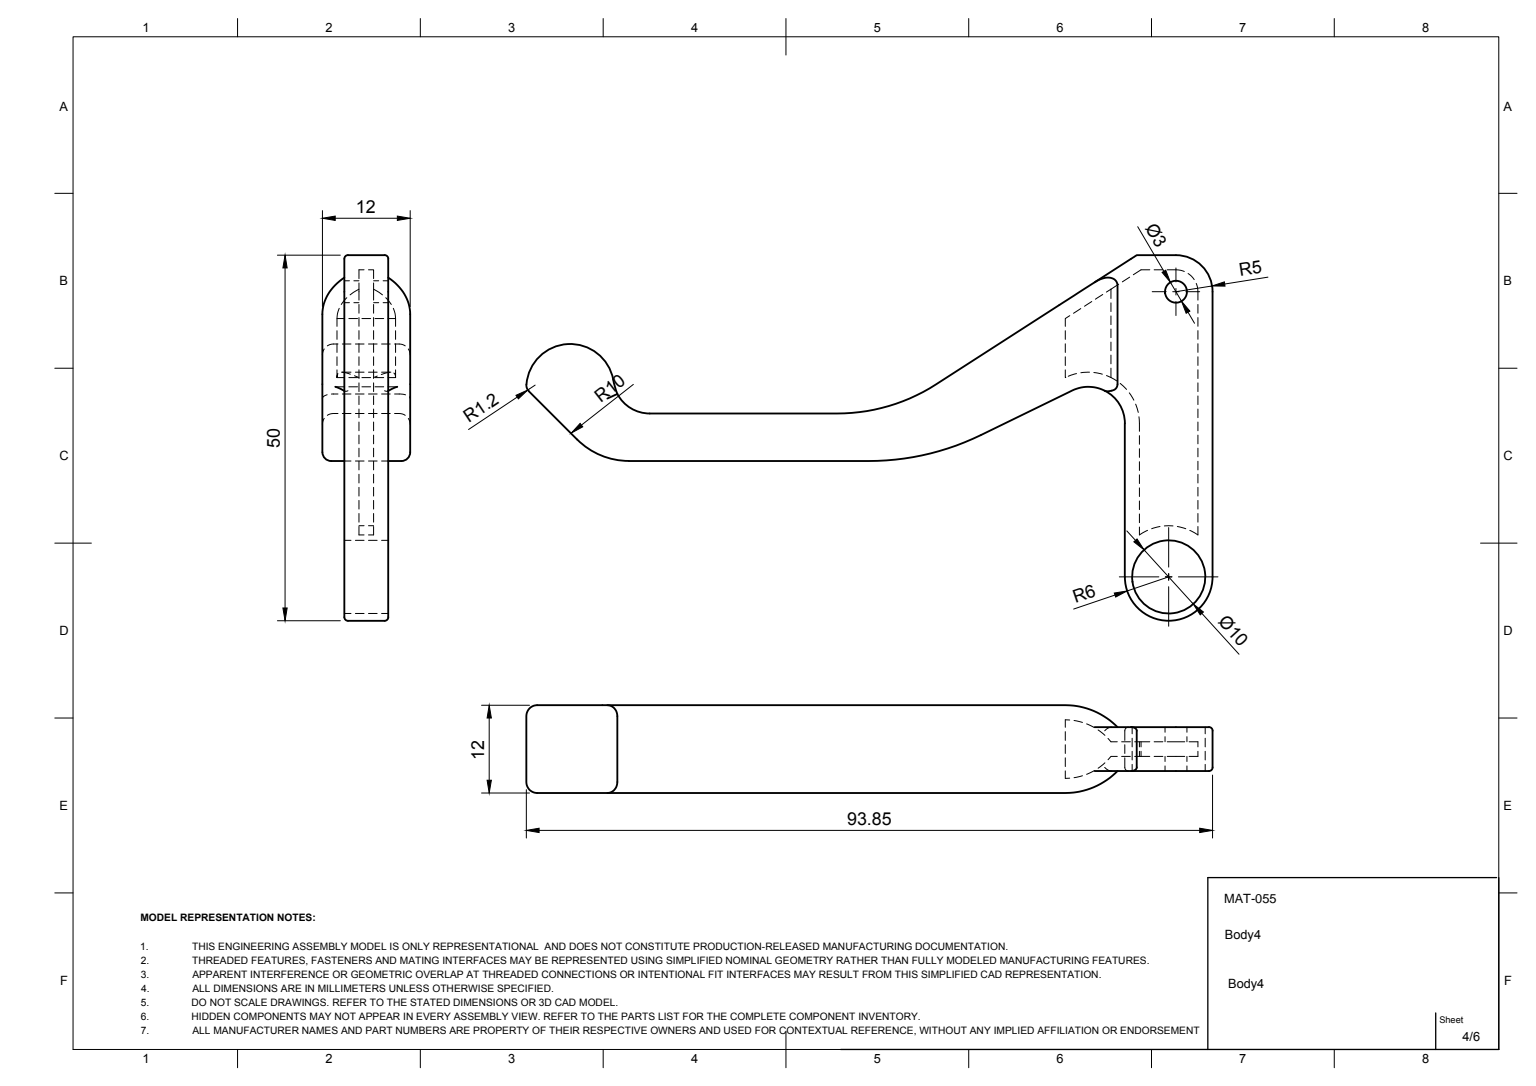
ISO-10303-21;
HEADER;
FILE_DESCRIPTION (('STEP AP214'),
    '1' );
FILE_NAME ('Body4.step',
    '2026-10-30T09:41:00',
    ( '' ),
    ( '' ),
    'SwSTEP 2.0',
    'SolidWorks 2020',
    '' );
FILE_SCHEMA (( 'AUTOMOTIVE_DESIGN' ));
ENDSEC;

DATA;
#3=ORIENTED_EDGE ( 'NONE', *, *, #32082, .F. ) ;
#28=DIRECTION ( 'NONE',  ( 0.000000000000000000, 0.000000000000000000, -1.000000000000000000 ) ) ;
#32=CARTESIAN_POINT ( 'NONE',  ( 74.32979735608419958, -48.45188957854135481, -10.89321520033831447 ) ) ;
#75=ORIENTED_EDGE ( 'NONE', *, *, #33478, .T. ) ;
#76=AXIS2_PLACEMENT_3D ( 'NONE', #7945, #18211, #24609 ) ;
#84=B_SPLINE_CURVE_WITH_KNOTS ( 'NONE', 3,
 ( #40412, #43376, #5506, #23076, #29462, #30146, #44061, #26048, #15786, #12373 ),
 .UNSPECIFIED., .F., .F.,
 ( 4, 2, 2, 2, 4 ),
 ( 0.000000000000000000, 0.0003215953659093761900, 0.0006431907318187523800, 0.0009647860977281285701, 0.001286381463637504760 ),
 .UNSPECIFIED. ) ;
#133=B_SPLINE_CURVE_WITH_KNOTS ( 'NONE', 3,
 ( #26160, #29806, #32757, #36631, #33206, #33421, #5174, #29130, #43042, #26387, #19321, #1981, #18865, #15907, #43720, #40297, #19544, #22961, #9061, #39624, #36853, #40065, #5622, #19092, #8163, #15001, #35960, #8830, #28914, #1530, #42824, #25494, #39398, #32977, #11810 ),
 .UNSPECIFIED., .F., .F.,
 ( 4, 2, 2, 1, 1, 2, 2, 1, 2, 2, 1, 1, 1, 1, 2, 2, 1, 1, 1, 1, 2, 2, 4 ),
 ( 0.000000000000000000, 0.06250000000002535472, 0.1250000000000507094, 0.1875000000000760503, 0.2187500000000859035, 0.2343750000000941469, 0.2500000000001023626, 0.3125000000001353362, 0.3281250000001413869, 0.3437500000001474376, 0.3750000000001494360, 0.4375000000001431633, 0.4687500000001400546, 0.4843750000001384448, 0.4921875000001327272, 0.5000000000001270095, 0.6250000000001643130, 0.6875000000001828537, 0.7187500000001921796, 0.7343750000001968425, 0.7421875000001944001, 0.7500000000001918465, 1.000000000000000000 ),
 .UNSPECIFIED. ) ;
#140=CARTESIAN_POINT ( 'NONE',  ( 63.90572062191856872, -12.84802420451643812, -16.01116961145836370 ) ) ;
#144=DIRECTION ( 'NONE',  ( 0.000000000000000000, 0.000000000000000000, -1.000000000000000000 ) ) ;
#154=CARTESIAN_POINT ( 'NONE',  ( 74.47157298427187300, -3.053873105668316601, -12.39321520033831447 ) ) ;
#166=VERTEX_POINT ( 'NONE', #36740 ) ;
#185=CYLINDRICAL_SURFACE ( 'NONE', #31797, 1.499999999999999556 ) ;
#188=( BOUNDED_CURVE ( )  B_SPLINE_CURVE ( 3, ( #13503, #13725, #28295, #3452 ),
 .UNSPECIFIED., .F., .F. ) 
 B_SPLINE_CURVE_WITH_KNOTS ( ( 4, 4 ),
 ( 4.712388980384689674, 4.721492906269370238 ),
 .UNSPECIFIED. ) 
 CURVE ( )  GEOMETRIC_REPRESENTATION_ITEM ( )  RATIONAL_B_SPLINE_CURVE ( ( 1.000000000000000000, 0.9999930932230500780, 0.9999930932230500780, 1.000000000000000000 ) ) 
 REPRESENTATION_ITEM ( '' )  );
#204=CARTESIAN_POINT ( 'NONE',  ( 70.47992290675011873, 2.032776587329049978, -16.39321520033831447 ) ) ;
#214=CARTESIAN_POINT ( 'NONE',  ( 64.04449450084898388, -15.08552066177155382, -16.37144510805424957 ) ) ;
#215=DIRECTION ( 'NONE',  ( -0.1352586133457950590, -0.9908103287288504424, 0.000000000000000000 ) ) ;
#226=DIRECTION ( 'NONE',  ( 0.000000000000000000, 0.000000000000000000, -1.000000000000000000 ) ) ;
#257=CARTESIAN_POINT ( 'NONE',  ( 64.46696884417693241, -15.35047623415474405, -15.89321305673442986 ) ) ;
#259=VERTEX_POINT ( 'NONE', #5961 ) ;
#276=EDGE_CURVE ( 'NONE', #36610, #20781, #19248, .T. ) ;
#291=CARTESIAN_POINT ( 'NONE',  ( 27.57768543387103222, -14.97172645945875935, -19.39321520033831447 ) ) ;
#293=ORIENTED_EDGE ( 'NONE', *, *, #35379, .F. ) ;
#305=CARTESIAN_POINT ( 'NONE',  ( 74.32979735608419958, -48.45188957854135481, -10.39321520033831625 ) ) ;
#312=ORIENTED_EDGE ( 'NONE', *, *, #19134, .T. ) ;
#326=AXIS2_PLACEMENT_3D ( 'NONE', #2034, #13672, #6599 ) ;
#349=AXIS2_PLACEMENT_3D ( 'NONE', #13047, #20117, #28 ) ;
#362=CARTESIAN_POINT ( 'NONE',  ( 61.78196040322745120, -12.46576002031727448, -17.04883285403948534 ) ) ;
#369=FACE_OUTER_BOUND ( 'NONE', #21979, .T. ) ;
#401=EDGE_CURVE ( 'NONE', #31742, #38280, #42421, .T. ) ;
#430=CIRCLE ( 'NONE', #37583, 1.200000000000000178 ) ;
#432=ORIENTED_EDGE ( 'NONE', *, *, #12226, .F. ) ;
#436=CARTESIAN_POINT ( 'NONE',  ( 62.89921056888596240, -13.37922507188889654, -18.73918694084264303 ) ) ;
#440=AXIS2_PLACEMENT_3D ( 'NONE', #42881, #38535, #14611 ) ;
#469=EDGE_CURVE ( 'NONE', #23752, #259, #6849, .T. ) ;
#472=DIRECTION ( 'NONE',  ( 0.000000000000000000, 0.000000000000000000, -1.000000000000000000 ) ) ;
#478=LINE ( 'NONE', #3232, #42202 ) ;
#490=EDGE_CURVE ( 'NONE', #13961, #15605, #188, .T. ) ;
#497=CARTESIAN_POINT ( 'NONE',  ( 64.24243542014160369, -41.01918285936451269, -16.39321520033831447 ) ) ;
#511=VERTEX_POINT ( 'NONE', #38315 ) ;
#512=AXIS2_PLACEMENT_3D ( 'NONE', #29324, #1497, #9256 ) ;
#522=EDGE_CURVE ( 'NONE', #12356, #39715, #34544, .T. ) ;
#531=DIRECTION ( 'NONE',  ( 0.000000000000000000, 0.000000000000000000, -1.000000000000000000 ) ) ;
#532=ADVANCED_FACE ( 'NONE', ( #3665 ), #7307, .T. ) ;
#553=DIRECTION ( 'NONE',  ( -0.6049664196031393493, 0.7962509850245451659, 0.000000000000000000 ) ) ;
#554=CARTESIAN_POINT ( 'NONE',  ( 62.74499803203641335, -14.59121584191781018, -17.38686684484656908 ) ) ;
#556=EDGE_LOOP ( 'NONE', ( #34925, #21880, #41263, #43526, #26990, #41505, #39389, #13719, #5501, #37121, #24239, #17991 ) ) ;
#560=CARTESIAN_POINT ( 'NONE',  ( 64.90995917204980969, -13.28308322077656278, -11.63059948780157349 ) ) ;
#584=DIRECTION ( 'NONE',  ( 0.000000000000000000, 0.000000000000000000, -1.000000000000000000 ) ) ;
#661=CARTESIAN_POINT ( 'NONE',  ( 64.65529483955577916, -15.48286765530762388, -15.65793769818279735 ) ) ;
#671=CARTESIAN_POINT ( 'NONE',  ( 27.57768543387103222, -14.97172645945875935, -19.39321520033831447 ) ) ;
#677=CARTESIAN_POINT ( 'NONE',  ( 61.14757329627086335, -2.318400467695852285, -17.89321520033712432 ) ) ;
#698=ORIENTED_EDGE ( 'NONE', *, *, #12294, .T. ) ;
#712=CARTESIAN_POINT ( 'NONE',  ( 63.70438564670760684, -13.53232477329181727, -18.38352350030624294 ) ) ;
#716=ORIENTED_EDGE ( 'NONE', *, *, #37812, .T. ) ;
#750=EDGE_LOOP ( 'NONE', ( #41830, #3198, #2175, #16810 ) ) ;
#764=CARTESIAN_POINT ( 'NONE',  ( 35.90261398037149121, 14.17005867477686820, -19.39321520033831447 ) ) ;
#772=CARTESIAN_POINT ( 'NONE',  ( 64.39654352178588681, -13.03842319615433709, -11.15581236813648935 ) ) ;
#788=EDGE_LOOP ( 'NONE', ( #32650, #7157 ) ) ;
#799=CARTESIAN_POINT ( 'NONE',  ( 64.46696884418977902, -15.35047623416358142, -10.89321734395795893 ) ) ;
#809=DIRECTION ( 'NONE',  ( -0.1352586133457901185, -0.9908103287288512195, 0.000000000000000000 ) ) ;
#810=AXIS2_PLACEMENT_3D ( 'NONE', #14418, #28328, #11900 ) ;
#812=CARTESIAN_POINT ( 'NONE',  ( 60.96717296766336602, -14.49347760901631688, -8.701126109306295930 ) ) ;
#854=VERTEX_POINT ( 'NONE', #33717 ) ;
#857=EDGE_CURVE ( 'NONE', #16139, #18111, #18527, .T. ) ;
#873=VERTEX_POINT ( 'NONE', #7043 ) ;
#880=CARTESIAN_POINT ( 'NONE',  ( 59.41476255453773803, -13.68180535374018092, -7.393215200338314474 ) ) ;
#898=DIRECTION ( 'NONE',  ( 0.000000000000000000, 0.000000000000000000, 1.000000000000000000 ) ) ;
#905=CARTESIAN_POINT ( 'NONE',  ( 61.98291279206183191, -3.705398587646214992, -19.39321520033831447 ) ) ;
#915=DIRECTION ( 'NONE',  ( 0.9908103287288504424, -0.1352586133457951423, 0.000000000000000000 ) ) ;
#932=CARTESIAN_POINT ( 'NONE',  ( -1.145390592550938447, -14.88589425535891841, -7.393215200338315363 ) ) ;
#938=EDGE_LOOP ( 'NONE', ( #22426, #35188, #1636, #40965 ) ) ;
#944=CARTESIAN_POINT ( 'NONE',  ( 66.31928500851137187, -14.71576354012722021, -16.39321520033831447 ) ) ;
#1006=CARTESIAN_POINT ( 'NONE',  ( -1.637506834317598026, -6.775152287193681566, -8.893215200338314474 ) ) ;
#1035=EDGE_CURVE ( 'NONE', #40192, #37616, #36694, .T. ) ;
#1037=CARTESIAN_POINT ( 'NONE',  ( 64.06711464991177252, -13.62989902061672431, -8.594543081115894267 ) ) ;
#1043=DIRECTION ( 'NONE',  ( 0.000000000000000000, 0.000000000000000000, -1.000000000000000000 ) ) ;
#1064=ADVANCED_FACE ( 'NONE', ( #14107 ), #43297, .T. ) ;
#1067=CARTESIAN_POINT ( 'NONE',  ( 65.10287265247757205, -0.4742552606671820992, -16.39321520033831447 ) ) ;
#1079=ORIENTED_EDGE ( 'NONE', *, *, #19134, .F. ) ;
#1083=CARTESIAN_POINT ( 'NONE',  ( 80.41643495664496299, -3.865424785743087899, -10.39321520033831625 ) ) ;
#1084=CARTESIAN_POINT ( 'NONE',  ( 64.05455464101120810, -2.913905561056498339, -7.947895114335570277 ) ) ;
#1111=CARTESIAN_POINT ( 'NONE',  ( 63.72671350766138687, -14.88170162854069645, -18.28103043643234571 ) ) ;
#1126=LINE ( 'NONE', #14821, #18340 ) ;
#1143=CARTESIAN_POINT ( 'NONE',  ( 53.69308256885118169, -7.449060273445263114, -7.393215200338315363 ) ) ;
#1144=DIRECTION ( 'NONE',  ( 0.1352586133457901185, 0.9908103287288512195, 0.000000000000000000 ) ) ;
#1145=VECTOR ( 'NONE', #26126, 999.9999999999998863 ) ;
#1153=ORIENTED_EDGE ( 'NONE', *, *, #29788, .T. ) ;
#1169=CIRCLE ( 'NONE', #19398, 10.00000000000000000 ) ;
#1173=ORIENTED_EDGE ( 'NONE', *, *, #20334, .T. ) ;
#1191=CARTESIAN_POINT ( 'NONE',  ( 64.46696884418977902, -15.35047623416358142, -10.89321734395795893 ) ) ;
#1195=ORIENTED_EDGE ( 'NONE', *, *, #29638, .F. ) ;
#1199=DIRECTION ( 'NONE',  ( 0.000000000000000000, 0.000000000000000000, 1.000000000000000000 ) ) ;
#1203=CARTESIAN_POINT ( 'NONE',  ( 0.04488520489200759078, -6.166763362545027327, -18.19321520033831519 ) ) ;
#1211=ORIENTED_EDGE ( 'NONE', *, *, #8860, .T. ) ;
#1213=DIRECTION ( 'NONE',  ( -0.1352586133457950590, -0.9908103287288504424, 0.000000000000000000 ) ) ;
#1228=ORIENTED_EDGE ( 'NONE', *, *, #14201, .T. ) ;
#1261=AXIS2_PLACEMENT_3D ( 'NONE', #32042, #144, #7420 ) ;
#1263=DIRECTION ( 'NONE',  ( 0.000000000000000000, 0.000000000000000000, 1.000000000000000000 ) ) ;
#1265=CARTESIAN_POINT ( 'NONE',  ( 62.93954589823548673, -14.63888995810886051, -9.517290379660753530 ) ) ;
#1283=CIRCLE ( 'NONE', #23133, 1.499999999999998002 ) ;
#1285=CARTESIAN_POINT ( 'NONE',  ( -13.48289411298945595, -4.891473392625994343, -19.20673326947127180 ) ) ;
#1292=ORIENTED_EDGE ( 'NONE', *, *, #34484, .F. ) ;
#1293=CARTESIAN_POINT ( 'NONE',  ( 80.41643495664496299, -3.865424785743087899, -10.89321520033831447 ) ) ;
#1308=CARTESIAN_POINT ( 'NONE',  ( -13.00275943959160685, -4.132914642980755282, -7.537981892864975109 ) ) ;
#1314=EDGE_CURVE ( 'NONE', #7942, #42460, #4050, .T. ) ;
#1317=CARTESIAN_POINT ( 'NONE',  ( 65.55689610126231059, -13.67296395165911704, -12.39321520033831447 ) ) ;
#1330=CARTESIAN_POINT ( 'NONE',  ( 59.24641515291911986, -13.72835195454734425, -7.393215200338315363 ) ) ;
#1343=FILL_AREA_STYLE_COLOUR ( '', #11399 ) ;
#1353=EDGE_LOOP ( 'NONE', ( #6893, #31759, #18475, #18995, #18699 ) ) ;
#1370=CARTESIAN_POINT ( 'NONE',  ( 59.36680634945873436, -12.84644995903807541, -9.393215200338314474 ) ) ;
#1376=ORIENTED_EDGE ( 'NONE', *, *, #23481, .F. ) ;
#1397=CARTESIAN_POINT ( 'NONE',  ( 75.95778847736514194, -3.256761025687008537, -10.39321520033831625 ) ) ;
#1405=ORIENTED_EDGE ( 'NONE', *, *, #32534, .F. ) ;
#1407=CARTESIAN_POINT ( 'NONE',  ( 75.95778847736514194, -3.256761025687008537, -15.89321520033831447 ) ) ;
#1415=DIRECTION ( 'NONE',  ( 0.000000000000000000, 0.000000000000000000, 1.000000000000000000 ) ) ;
#1417=ORIENTED_EDGE ( 'NONE', *, *, #29638, .T. ) ;
#1426=DIRECTION ( 'NONE',  ( 0.000000000000000000, 0.000000000000000000, 1.000000000000000000 ) ) ;
#1427=ORIENTED_EDGE ( 'NONE', *, *, #41467, .F. ) ;
#1446=AXIS2_PLACEMENT_3D ( 'NONE', #14470, #25412, #11053 ) ;
#1469=VECTOR ( 'NONE', #21811, 1000.000000000000114 ) ;
#1483=CARTESIAN_POINT ( 'NONE',  ( 65.55342193993762123, -16.16218099987542800, -9.830679638262655118 ) ) ;
#1488=CARTESIAN_POINT ( 'NONE',  ( 66.31928500851137187, -14.71576354012722021, -10.39321520033831625 ) ) ;
#1497=DIRECTION ( 'NONE',  ( 0.000000000000000000, 0.000000000000000000, -1.000000000000000000 ) ) ;
#1498=VECTOR ( 'NONE', #3951, 1000.000000000000000 ) ;
#1527=CARTESIAN_POINT ( 'NONE',  ( 68.14371629974728251, -1.351251493923715685, -10.39321520033831625 ) ) ;
#1530=CARTESIAN_POINT ( 'NONE',  ( 66.05753635973103144, -0.1399854074271419946, -16.39321520033832158 ) ) ;
#1571=FACE_OUTER_BOUND ( 'NONE', #24276, .T. ) ;
#1591=CARTESIAN_POINT ( 'NONE',  ( 66.31928500851137187, -14.71576354012722021, -16.39321520033831447 ) ) ;
#1611=EDGE_LOOP ( 'NONE', ( #21835, #10008, #36290, #40632 ) ) ;
#1620=ORIENTED_EDGE ( 'NONE', *, *, #9988, .T. ) ;
#1626=VERTEX_POINT ( 'NONE', #1984 ) ;
#1632=CIRCLE ( 'NONE', #25668, 7.000000000000000888 ) ;
#1636=ORIENTED_EDGE ( 'NONE', *, *, #10913, .F. ) ;
#1667=CARTESIAN_POINT ( 'NONE',  ( -2.527712056240301930, -7.043022739214354289, -7.506402576757856160 ) ) ;
#1683=ORIENTED_EDGE ( 'NONE', *, *, #31150, .F. ) ;
#1687=AXIS2_PLACEMENT_3D ( 'NONE', #22360, #36254, #7999 ) ;
#1705=LINE ( 'NONE', #25445, #8559 ) ;
#1706=CARTESIAN_POINT ( 'NONE',  ( 66.18166293637838749, -0.1100759832042771530, -10.39321520033831625 ) ) ;
#1707=CARTESIAN_POINT ( 'NONE',  ( -1.923444331009816155, -6.861511549474196947, -18.79244370401574216 ) ) ;
#1708=CARTESIAN_POINT ( 'NONE',  ( 65.24959551893836363, -14.08404458135745152, -9.384265616240702101 ) ) ;
#1722=DIRECTION ( 'NONE',  ( 0.9498278979187094739, 0.3127730236694427068, -0.000000000000000000 ) ) ;
#1747=CLOSED_SHELL ( 'NONE', ( #4152, #37866, #40832, #17245, #16199, #21143, #36527, #26583, #23655, #20308, #38149, #18533, #35581, #9060, #4115, #13887, #44627, #15699, #28669, #35867, #21510, #34238, #35882, #34304, #5814, #38233, #42050, #33081, #39264, #10525, #29766, #20277, #13735, #40925, #19555, #43598, #6488, #4374, #15680, #7071, #24586, #1064, #38417, #19728, #39940, #41099, #4945, #44561, #38547, #4966, #20625, #26823, #10638, #12784, #14728, #37236, #36466, #14740, #3572, #33654, #43377, #17043, #18627, #23403, #28076, #37922, #4151, #25624, #14144, #30621, #36573, #2068, #37329, #6478, #6539, #28402, #39232, #44240, #532, #16742, #12305, #32549, #31783, #4091, #35680 ) ) ;
#1795=VERTEX_POINT ( 'NONE', #41877 ) ;
#1833=VECTOR ( 'NONE', #22228, 1000.000000000000000 ) ;
#1884=CARTESIAN_POINT ( 'NONE',  ( 62.60955873541980310, -3.465946903308488647, -19.20240821814916288 ) ) ;
#1885=CARTESIAN_POINT ( 'NONE',  ( -6.962123463324031647, -11.49046785505262136, -19.39321520033831447 ) ) ;
#1912=( BOUNDED_CURVE ( )  B_SPLINE_CURVE ( 3, ( #16184, #40122, #36238, #36461 ),
 .UNSPECIFIED., .F., .F. ) 
 B_SPLINE_CURVE_WITH_KNOTS ( ( 4, 4 ),
 ( 4.664242276651448194, 4.712388980384689674 ),
 .UNSPECIFIED. ) 
 CURVE ( )  GEOMETRIC_REPRESENTATION_ITEM ( )  RATIONAL_B_SPLINE_CURVE ( ( 1.000000000000000000, 0.9998068339056410680, 0.9998068339056410680, 1.000000000000000000 ) ) 
 REPRESENTATION_ITEM ( '' )  );
#1950=CARTESIAN_POINT ( 'NONE',  ( -13.78505786413266243, -3.796669003528118758, -18.12937505555870388 ) ) ;
#1964=CYLINDRICAL_SURFACE ( 'NONE', #9953, 4.999999999999997335 ) ;
#1972=VERTEX_POINT ( 'NONE', #3772 ) ;
#1978=CARTESIAN_POINT ( 'NONE',  ( 62.64330450333520162, -3.453051920597017155, -7.590354665846188453 ) ) ;
#1981=CARTESIAN_POINT ( 'NONE',  ( 67.79734085828376067, -0.4026402971269220643, -16.39321520033831447 ) ) ;
#1984=CARTESIAN_POINT ( 'NONE',  ( 76.63408154409412987, 1.697290617957241565, -10.89321520033831447 ) ) ;
#1993=EDGE_CURVE ( 'NONE', #43140, #12130, #45032, .T. ) ;
#2003=CARTESIAN_POINT ( 'NONE',  ( -12.36826994950264336, -4.374949827406453551, -7.393215200338315363 ) ) ;
#2034=CARTESIAN_POINT ( 'NONE',  ( -1.145390592550938447, -14.88589425535891841, -8.593215200338315540 ) ) ;
#2048=ORIENTED_EDGE ( 'NONE', *, *, #29511, .T. ) ;
#2056=VERTEX_POINT ( 'NONE', #24984 ) ;
#2068=ADVANCED_FACE ( 'NONE', ( #28193 ), #12743, .T. ) ;
#2083=ORIENTED_EDGE ( 'NONE', *, *, #25009, .F. ) ;
#2109=CARTESIAN_POINT ( 'NONE',  ( 62.59689981967161998, -3.470785003659166090, -19.20476018416520958 ) ) ;
#2128=VERTEX_POINT ( 'NONE', #24757 ) ;
#2147=EDGE_CURVE ( 'NONE', #24167, #2128, #34986, .T. ) ;
#2148=CARTESIAN_POINT ( 'NONE',  ( 68.16708570727516303, -1.180063502400580999, -10.39321520033831625 ) ) ;
#2153=ORIENTED_EDGE ( 'NONE', *, *, #14241, .F. ) ;
#2156=CARTESIAN_POINT ( 'NONE',  ( 65.41257106814472877, -15.47412461924279725, -10.39321520033831625 ) ) ;
#2165=FACE_OUTER_BOUND ( 'NONE', #28094, .T. ) ;
#2168=CARTESIAN_POINT ( 'NONE',  ( -13.77941350934472808, -4.501197414032524158, -18.63512858394170379 ) ) ;
#2175=ORIENTED_EDGE ( 'NONE', *, *, #19187, .F. ) ;
#2183=ORIENTED_EDGE ( 'NONE', *, *, #32555, .T. ) ;
#2187=EDGE_CURVE ( 'NONE', #4486, #33968, #12023, .T. ) ;
#2200=CARTESIAN_POINT ( 'NONE',  ( -1.932019669644797988, -4.762702382056356321, -17.89321520033831447 ) ) ;
#2232=CARTESIAN_POINT ( 'NONE',  ( -12.36826994950264513, -4.374949827406456215, -19.39321520033831447 ) ) ;
#2239=DIRECTION ( 'NONE',  ( 0.9063289528979890930, 0.4225728684367167087, 0.000000000000000000 ) ) ;
#2263=DIRECTION ( 'NONE',  ( -0.9908103287288503314, 0.1352586133457950868, 0.000000000000000000 ) ) ;
#2271=ORIENTED_EDGE ( 'NONE', *, *, #12226, .T. ) ;
#2343=ORIENTED_EDGE ( 'NONE', *, *, #857, .F. ) ;
#2344=CARTESIAN_POINT ( 'NONE',  ( -2.588851517412736669, -7.061334938601206979, -7.481563165383908753 ) ) ;
#2355=VECTOR ( 'NONE', #41919, 1000.000000000000000 ) ;
#2376=ORIENTED_EDGE ( 'NONE', *, *, #6085, .T. ) ;
#2388=CARTESIAN_POINT ( 'NONE',  ( 74.82520252044861309, -48.51951888521425360, -16.39321520033831447 ) ) ;
#2399=FACE_OUTER_BOUND ( 'NONE', #27872, .T. ) ;
#2440=EDGE_CURVE ( 'NONE', #5770, #22762, #42644, .T. ) ;
#2464=ORIENTED_EDGE ( 'NONE', *, *, #34499, .F. ) ;
#2490=DIRECTION ( 'NONE',  ( 0.9498278979187092519, 0.3127730236694430399, -0.000000000000000000 ) ) ;
#2509=CARTESIAN_POINT ( 'NONE',  ( -3.429934629567074733, -4.841764211284793618, -19.39321520033831447 ) ) ;
#2573=CARTESIAN_POINT ( 'NONE',  ( -2.615402842485104351, -7.069279208319384722, -7.472031487140878170 ) ) ;
#2590=AXIS2_PLACEMENT_3D ( 'NONE', #14721, #584, #27744 ) ;
#2595=AXIS2_PLACEMENT_3D ( 'NONE', #30427, #27464, #13777 ) ;
#2598=CARTESIAN_POINT ( 'NONE',  ( 60.11760374155740294, -14.70486118635416695, -7.429569208445770734 ) ) ;
#2605=DIRECTION ( 'NONE',  ( -0.9063289528979890930, -0.4225728684367167087, 0.000000000000000000 ) ) ;
#2608=DIRECTION ( 'NONE',  ( 0.000000000000000000, 0.000000000000000000, 1.000000000000000000 ) ) ;
#2615=FACE_OUTER_BOUND ( 'NONE', #42287, .T. ) ;
#2622=DIRECTION ( 'NONE',  ( -0.9908103287288504424, 0.1352586133457950313, 0.000000000000000000 ) ) ;
#2631=STYLED_ITEM ( 'NONE', ( #35992 ), #43323 ) ;
#2652=CARTESIAN_POINT ( 'NONE',  ( 71.62928943233082180, 0.3619606153155430217, -12.39321520033831447 ) ) ;
#2665=ORIENTED_EDGE ( 'NONE', *, *, #4911, .T. ) ;
#2707=DIRECTION ( 'NONE',  ( -0.9908103287288504424, 0.1352586133457950313, 0.000000000000000000 ) ) ;
#2714=LINE ( 'NONE', #30534, #38940 ) ;
#2749=VECTOR ( 'NONE', #7883, 1000.000000000000000 ) ;
#2755=ORIENTED_EDGE ( 'NONE', *, *, #6941, .T. ) ;
#2760=EDGE_LOOP ( 'NONE', ( #31215, #432, #27283, #35161 ) ) ;
#2773=DIRECTION ( 'NONE',  ( 0.000000000000000000, 0.000000000000000000, 1.000000000000000000 ) ) ;
#2786=CARTESIAN_POINT ( 'NONE',  ( 46.47434218039879283, -17.93412427487546523, -8.593215200338315540 ) ) ;
#2787=FACE_OUTER_BOUND ( 'NONE', #19625, .T. ) ;
#2803=ORIENTED_EDGE ( 'NONE', *, *, #25009, .T. ) ;
#2818=VERTEX_POINT ( 'NONE', #291 ) ;
#2850=DIRECTION ( 'NONE',  ( 0.3127730236694482580, -0.9498278979187074755, 0.000000000000000000 ) ) ;
#2852=DIRECTION ( 'NONE',  ( -0.000000000000000000, -0.000000000000000000, 1.000000000000000000 ) ) ;
#2856=CARTESIAN_POINT ( 'NONE',  ( 31.16203868753470019, 11.28474725185576055, -17.89321520033831447 ) ) ;
#2883=CARTESIAN_POINT ( 'NONE',  ( 66.07656475110815109, -2.141145020708993929, -8.744744089885024607 ) ) ;
#2925=AXIS2_PLACEMENT_3D ( 'NONE', #18987, #8724, #11703 ) ;
#2926=CARTESIAN_POINT ( 'NONE',  ( 61.63318325272354770, -19.46990085680238636, -15.89321520033831447 ) ) ;
#2979=DIRECTION ( 'NONE',  ( 0.000000000000000000, 0.000000000000000000, 1.000000000000000000 ) ) ;
#2987=VERTEX_POINT ( 'NONE', #17847 ) ;
#2990=CARTESIAN_POINT ( 'NONE',  ( 61.36049780884140148, -12.47513267055688502, -9.628222199120516578 ) ) ;
#2994=EDGE_CURVE ( 'NONE', #9021, #11150, #41201, .T. ) ;
#2996=EDGE_LOOP ( 'NONE', ( #25071, #25421, #35320, #36704, #2153 ) ) ;
#3010=DIRECTION ( 'NONE',  ( -0.9908103287288505534, 0.1352586133457950035, 0.000000000000000000 ) ) ;
#3046=CIRCLE ( 'NONE', #31438, 26.50000000000000000 ) ;
#3110=CARTESIAN_POINT ( 'NONE',  ( 67.28387040543748299, -1.679813135375296529, -9.537078095872010053 ) ) ;
#3183=VERTEX_POINT ( 'NONE', #42918 ) ;
#3198=ORIENTED_EDGE ( 'NONE', *, *, #522, .F. ) ;
#3222=DIRECTION ( 'NONE',  ( 0.000000000000000000, 0.000000000000000000, 1.000000000000000000 ) ) ;
#3232=CARTESIAN_POINT ( 'NONE',  ( 66.58723489636778936, -20.14619392353143112, -19.39321520033831447 ) ) ;
#3242=ORIENTED_EDGE ( 'NONE', *, *, #6941, .F. ) ;
#3254=CARTESIAN_POINT ( 'NONE',  ( 77.44400397045842510, -3.459648945705700473, -14.39321520033831625 ) ) ;
#3269=ORIENTED_EDGE ( 'NONE', *, *, #25124, .T. ) ;
#3279=CARTESIAN_POINT ( 'NONE',  ( 63.09505974864278244, -3.280483143683338820, -7.685112946281191348 ) ) ;
#3291=CARTESIAN_POINT ( 'NONE',  ( -3.049772195457630897, -7.199189612102626867, -19.39321520033830737 ) ) ;
#3340=CARTESIAN_POINT ( 'NONE',  ( 70.47992290675011873, 2.032776587329049978, -10.39321520033831625 ) ) ;
#3342=CARTESIAN_POINT ( 'NONE',  ( 61.06105367438289733, -12.49321934622164321, -17.22529996229299343 ) ) ;
#3348=DIRECTION ( 'NONE',  ( 0.000000000000000000, 0.000000000000000000, 1.000000000000000000 ) ) ;
#3370=DIRECTION ( 'NONE',  ( -0.000000000000000000, -0.000000000000000000, 1.000000000000000000 ) ) ;
#3373=ORIENTED_EDGE ( 'NONE', *, *, #39824, .F. ) ;
#3386=VERTEX_POINT ( 'NONE', #34336 ) ;
#3388=AXIS2_PLACEMENT_3D ( 'NONE', #28349, #7591, #31979 ) ;
#3389=DIRECTION ( 'NONE',  ( 0.000000000000000000, 0.000000000000000000, 1.000000000000000000 ) ) ;
#3393=CARTESIAN_POINT ( 'NONE',  ( -13.78505786849335379, -3.796669023459796843, -8.893215200338350002 ) ) ;
#3435=AXIS2_PLACEMENT_3D ( 'NONE', #1407, #18297, #4828 ) ;
#3452=CARTESIAN_POINT ( 'NONE',  ( 59.44377208703740223, -12.82110557137145967, -17.39288367676203606 ) ) ;
#3455=DIRECTION ( 'NONE',  ( 0.000000000000000000, 0.000000000000000000, -1.000000000000000000 ) ) ;
#3501=FACE_OUTER_BOUND ( 'NONE', #32187, .T. ) ;
#3548=CARTESIAN_POINT ( 'NONE',  ( 65.70869026611384811, -0.1917948075113792838, -10.71553487254586656 ) ) ;
#3554=CYLINDRICAL_SURFACE ( 'NONE', #2590, 1.499999999999998002 ) ;
#3557=CARTESIAN_POINT ( 'NONE',  ( 63.16361418624702395, -12.63457483197140085, -16.47427386053546527 ) ) ;
#3562=CYLINDRICAL_SURFACE ( 'NONE', #26727, 1.199999999999996625 ) ;
#3568=DIRECTION ( 'NONE',  ( 0.000000000000000000, 0.000000000000000000, -1.000000000000000000 ) ) ;
#3572=ADVANCED_FACE ( 'NONE', ( #11749 ), #21101, .F. ) ;
#3632=CARTESIAN_POINT ( 'NONE',  ( 63.78480611294602909, -13.55202615601718463, -18.34317296867338598 ) ) ;
#3645=FACE_OUTER_BOUND ( 'NONE', #37899, .T. ) ;
#3663=VECTOR ( 'NONE', #42879, 1000.000000000000000 ) ;
#3665=FACE_OUTER_BOUND ( 'NONE', #19411, .T. ) ;
#3668=CARTESIAN_POINT ( 'NONE',  ( 76.56645223742121686, 1.201885453592819397, -10.89321520033831447 ) ) ;
#3676=EDGE_CURVE ( 'NONE', #43140, #23633, #26628, .T. ) ;
#3718=DIRECTION ( 'NONE',  ( -0.9908103287288504424, 0.1352586133457951423, 0.000000000000000000 ) ) ;
#3739=CARTESIAN_POINT ( 'NONE',  ( 63.28220228970403127, -14.74607418324612418, -17.03279905538827066 ) ) ;
#3756=VECTOR ( 'NONE', #13524, 1000.000000000000000 ) ;
#3760=ORIENTED_EDGE ( 'NONE', *, *, #13500, .T. ) ;
#3772=CARTESIAN_POINT ( 'NONE',  ( 76.56645223742121686, 1.201885453592819397, -16.39321520033831447 ) ) ;
#3812=VECTOR ( 'NONE', #10685, 1000.000000000000000 ) ;
#3828=B_SPLINE_CURVE_WITH_KNOTS ( 'NONE', 3,
 ( #11759, #25669, #39574, #18818, #22237, #36357, #1707, #26112, #11988, #25889, #32709, #39794, #5128, #19045, #15630, #29534, #43450, #40018, #22688, #36586, #5361, #27477, #33841, #41396, #30213, #43901, #9694, #3291, #37032 ),
 .UNSPECIFIED., .F., .F.,
 ( 4, 2, 2, 2, 1, 1, 2, 2, 2, 2, 1, 1, 1, 2, 2, 2, 4 ),
 ( 0.000000000000000000, 0.2500000000000469624, 0.3750000000000684452, 0.4375000000000791589, 0.4687500000000845435, 0.4843750000000872080, 0.4921875000000887623, 0.5000000000000902611, 0.6250000000000713873, 0.6875000000000619504, 0.7187500000000581757, 0.7343750000000563993, 0.7421875000000554001, 0.7460937500000548450, 0.7500000000000544009, 0.8750000000000272005, 1.000000000000000000 ),
 .UNSPECIFIED. ) ;
#3830=CARTESIAN_POINT ( 'NONE',  ( 75.95778847736514194, -3.256761025687008537, -10.89321520033831447 ) ) ;
#3854=PLANE ( 'NONE',  #8272 ) ;
#3868=AXIS2_PLACEMENT_3D ( 'NONE', #37031, #2608, #12668 ) ;
#3869=EDGE_CURVE ( 'NONE', #12923, #2818, #28104, .T. ) ;
#3886=DIRECTION ( 'NONE',  ( -0.6049664196031392382, 0.7962509850245451659, 0.000000000000000000 ) ) ;
#3897=MECHANICAL_DESIGN_GEOMETRIC_PRESENTATION_REPRESENTATION('',(#25756),#36635);
#3898=DIRECTION ( 'NONE',  ( -0.9908103287288504424, 0.1352586133457950590, 0.000000000000000000 ) ) ;
#3900=AXIS2_PLACEMENT_3D ( 'NONE', #13422, #23911, #30507 ) ;
#3939=ORIENTED_EDGE ( 'NONE', *, *, #36160, .T. ) ;
#3951=DIRECTION ( 'NONE',  ( -0.9908103287288505534, 0.1352586133457944206, 0.000000000000000000 ) ) ;
#3969=CARTESIAN_POINT ( 'NONE',  ( 65.03532339491583514, -13.35226529162342501, -11.76448087493823280 ) ) ;
#3979=CARTESIAN_POINT ( 'NONE',  ( 54.86886719809545809, -45.79521720516596872, -9.393215200338314474 ) ) ;
#3982=VERTEX_POINT ( 'NONE', #6256 ) ;
#3989=CARTESIAN_POINT ( 'NONE',  ( 60.45894907855897316, -4.846173528048923096, -17.39321520033831447 ) ) ;
#3996=CARTESIAN_POINT ( 'NONE',  ( 62.56397285973651634, -12.53174821361586488, -16.75792485075395533 ) ) ;
#4050=LINE ( 'NONE', #14552, #35258 ) ;
#4091=ADVANCED_FACE ( 'NONE', ( #17201 ), #10993, .T. ) ;
#4092=DIRECTION ( 'NONE',  ( -0.9908103287288503314, 0.1352586133457958362, 0.000000000000000000 ) ) ;
#4107=CARTESIAN_POINT ( 'NONE',  ( 69.69189222815028018, -41.76310523276638520, -10.39321520033831625 ) ) ;
#4115=ADVANCED_FACE ( 'NONE', ( #3501 ), #13551, .T. ) ;
#4151=ADVANCED_FACE ( 'NONE', ( #40928 ), #23597, .F. ) ;
#4152=ADVANCED_FACE ( 'NONE', ( #31760 ), #17638, .F. ) ;
#4153=CARTESIAN_POINT ( 'NONE',  ( 31.16203868753470019, 11.28474725185576055, -7.393215200338315363 ) ) ;
#4167=ORIENTED_EDGE ( 'NONE', *, *, #42868, .F. ) ;
#4189=CARTESIAN_POINT ( 'NONE',  ( 61.41189896420279837, -3.923951091603942398, -19.36498282264282977 ) ) ;
#4210=CIRCLE ( 'NONE', #13702, 0.5000000000000004441 ) ;
#4228=FACE_OUTER_BOUND ( 'NONE', #43371, .T. ) ;
#4230=CARTESIAN_POINT ( 'NONE',  ( 62.22094884293999684, -14.48605613577975681, -7.865232863873874436 ) ) ;
#4236=CYLINDRICAL_SURFACE ( 'NONE', #29693, 8.000000000000000000 ) ;
#4240=EDGE_CURVE ( 'NONE', #17567, #15954, #18311, .T. ) ;
#4258=EDGE_CURVE ( 'NONE', #31347, #23752, #21505, .T. ) ;
#4273=CARTESIAN_POINT ( 'NONE',  ( -13.35201667389344315, -5.063733019641336597, -8.593215170849799023 ) ) ;
#4297=CARTESIAN_POINT ( 'NONE',  ( 75.95778847736514194, -3.256761025687008537, -15.89321520033831447 ) ) ;
#4301=CARTESIAN_POINT ( 'NONE',  ( 62.73786426684350204, -14.56780133514543607, -18.73718775869126318 ) ) ;
#4315=DIRECTION ( 'NONE',  ( -0.9908103287288504424, 0.1352586133457950590, 0.000000000000000000 ) ) ;
#4329=AXIS2_PLACEMENT_3D ( 'NONE', #27418, #40644, #20352 ) ;
#4343=CARTESIAN_POINT ( 'NONE',  ( 65.22669769703878728, -15.48412439713661648, -16.39321520033832513 ) ) ;
#4348=DIRECTION ( 'NONE',  ( -0.9908103287288503314, 0.1352586133457956419, 0.000000000000000000 ) ) ;
#4374=ADVANCED_FACE ( 'NONE', ( #18086 ), #31048, .T. ) ;
#4426=CARTESIAN_POINT ( 'NONE',  ( 63.41431291788855873, -12.69930909095325511, -10.45796961699282690 ) ) ;
#4434=ORIENTED_EDGE ( 'NONE', *, *, #42420, .T. ) ;
#4447=CARTESIAN_POINT ( 'NONE',  ( 60.45894907855897316, -4.846173528048923096, -9.393215200338314474 ) ) ;
#4454=EDGE_CURVE ( 'NONE', #16401, #39949, #1169, .T. ) ;
#4461=CARTESIAN_POINT ( 'NONE',  ( 63.72678816918493538, -14.88173340316315674, -8.505439947836993753 ) ) ;
#4486=VERTEX_POINT ( 'NONE', #20062 ) ;
#4490=SHAPE_DEFINITION_REPRESENTATION ( #14670, #30918 ) ;
#4505=CARTESIAN_POINT ( 'NONE',  ( 66.00964506737828685, -2.167441154595251440, -8.806695022995075561 ) ) ;
#4525=DIRECTION ( 'NONE',  ( 0.000000000000000000, 0.000000000000000000, -1.000000000000000000 ) ) ;
#4532=CARTESIAN_POINT ( 'NONE',  ( 60.62025573688512736, -14.54431086544325247, -19.30358038137204701 ) ) ;
#4542=PLANE ( 'NONE',  #35390 ) ;
#4547=CARTESIAN_POINT ( 'NONE',  ( 67.28358753636723577, -1.679921224420888981, -17.24955508517946967 ) ) ;
#4548=ORIENTED_EDGE ( 'NONE', *, *, #18053, .T. ) ;
#4584=CARTESIAN_POINT ( 'NONE',  ( 65.24959551893836363, -14.08404458135744797, -17.40216478443592507 ) ) ;
#4592=CIRCLE ( 'NONE', #1687, 4.999999999999997335 ) ;
#4613=CARTESIAN_POINT ( 'NONE',  ( 3.060777270043529619, -5.064559853354640317, -8.893215200338314474 ) ) ;
#4623=DIRECTION ( 'NONE',  ( 0.000000000000000000, 0.000000000000000000, -1.000000000000000000 ) ) ;
#4638=DIRECTION ( 'NONE',  ( 0.000000000000000000, 0.000000000000000000, 1.000000000000000000 ) ) ;
#4664=CARTESIAN_POINT ( 'NONE',  ( 60.06931813437629586, -14.72076136720887085, -8.603412892520118760 ) ) ;
#4665=DIRECTION ( 'NONE',  ( 0.9908103287288504424, -0.1352586133457949757, 0.000000000000000000 ) ) ;
#4672=CARTESIAN_POINT ( 'NONE',  ( -13.74784922440762713, -3.813634959067930819, -8.495864720811209025 ) ) ;
#4678=CARTESIAN_POINT ( 'NONE',  ( 66.01387875770896585, -14.50705293059987788, -10.06447537375617252 ) ) ;
#4707=EDGE_LOOP ( 'NONE', ( #16154, #4167, #4930, #15408 ) ) ;
#4744=VERTEX_POINT ( 'NONE', #15891 ) ;
#4755=EDGE_CURVE ( 'NONE', #31560, #2818, #7969, .T. ) ;
#4756=CARTESIAN_POINT ( 'NONE',  ( 55.68041887817022939, -39.85035523279287162, -17.39321520033831447 ) ) ;
#4763=SHAPE_REPRESENTATION_RELATIONSHIP ( 'NONE' , 'NONE' ,  #30918, #43323 ) ;
#4773=EDGE_LOOP ( 'NONE', ( #8065, #43824, #9275, #22865, #23073, #33451 ) ) ;
#4787=DIRECTION ( 'NONE',  ( 1.000000000000000000, 0.000000000000000000, 0.000000000000000000 ) ) ;
#4788=DIRECTION ( 'NONE',  ( -0.9908103287288504424, 0.1352586133457950590, 0.000000000000000000 ) ) ;
#4795=ORIENTED_EDGE ( 'NONE', *, *, #23426, .F. ) ;
#4828=DIRECTION ( 'NONE',  ( 0.9908103287288504424, -0.1352586133457951423, 0.000000000000000000 ) ) ;
#4832=AXIS2_PLACEMENT_3D ( 'NONE', #37080, #13836, #6777 ) ;
#4834=ORIENTED_EDGE ( 'NONE', *, *, #2994, .T. ) ;
#4845=EDGE_CURVE ( 'NONE', #35887, #24167, #34676, .T. ) ;
#4851=DIRECTION ( 'NONE',  ( 0.9908103287288504424, -0.1352586133457952533, 0.000000000000000000 ) ) ;
#4855=CARTESIAN_POINT ( 'NONE',  ( 27.78057335388972504, -13.48551096636548330, -19.39321520033831447 ) ) ;
#4885=ORIENTED_EDGE ( 'NONE', *, *, #33887, .T. ) ;
#4892=LINE ( 'NONE', #43891, #29240 ) ;
#4903=CARTESIAN_POINT ( 'NONE',  ( 59.75121349346655109, -13.58877957849837692, -7.404803486908546617 ) ) ;
#4911=EDGE_CURVE ( 'NONE', #11410, #23361, #23047, .T. ) ;
#4930=ORIENTED_EDGE ( 'NONE', *, *, #14554, .F. ) ;
#4943=EDGE_CURVE ( 'NONE', #2128, #10182, #40530, .T. ) ;
#4945=ADVANCED_FACE ( 'NONE', ( #28730 ), #4542, .F. ) ;
#4949=CARTESIAN_POINT ( 'NONE',  ( -13.43092278348643376, -3.953837739881414848, -7.878202387284918728 ) ) ;
#4966=ADVANCED_FACE ( 'NONE', ( #21878 ), #1964, .T. ) ;
#4977=EDGE_LOOP ( 'NONE', ( #14039, #7606, #8265, #14143 ) ) ;
#5061=EDGE_CURVE ( 'NONE', #32385, #9071, #1912, .T. ) ;
#5070=CYLINDRICAL_SURFACE ( 'NONE', #2925, 35.00000000000000711 ) ;
#5071=EDGE_LOOP ( 'NONE', ( #42487, #7890, #19368, #16058 ) ) ;
#5086=CARTESIAN_POINT ( 'NONE',  ( 67.69800074041313565, -1.521566938544754999, -16.82025522485820446 ) ) ;
#5113=DIRECTION ( 'NONE',  ( 1.000000000000000000, 0.000000000000000000, 0.000000000000000000 ) ) ;
#5116=CARTESIAN_POINT ( 'NONE',  ( 65.52504830115719869, -2.484121567297625788, -16.32284768336232261 ) ) ;
#5128=CARTESIAN_POINT ( 'NONE',  ( -2.055500662264778011, -6.901212958611610659, -18.95048905933739292 ) ) ;
#5129=CARTESIAN_POINT ( 'NONE',  ( 63.13224612813447578, -13.41522658373937915, -8.141029825667127184 ) ) ;
#5133=EDGE_LOOP ( 'NONE', ( #40422, #35648, #18943, #41192 ) ) ;
#5147=CARTESIAN_POINT ( 'NONE',  ( -13.83992782281680078, -4.421549056456191451, -18.43133312422856562 ) ) ;
#5154=ORIENTED_EDGE ( 'NONE', *, *, #41746, .F. ) ;
#5155=DIRECTION ( 'NONE',  ( -0.1352586133458019424, -0.9908103287288495542, 0.000000000000000000 ) ) ;
#5174=CARTESIAN_POINT ( 'NONE',  ( 68.03116533996660564, -0.6815855639037916580, -16.39321520033830737 ) ) ;
#5184=ORIENTED_EDGE ( 'NONE', *, *, #36160, .F. ) ;
#5197=CARTESIAN_POINT ( 'NONE',  ( 74.47157298427187300, -3.053873105668316601, -14.39321520033831625 ) ) ;
#5227=CARTESIAN_POINT ( 'NONE',  ( -3.429934629567074733, -4.841764211284793618, -8.893215200338314474 ) ) ;
#5288=CIRCLE ( 'NONE', #30780, 1.499999999999998002 ) ;
#5301=CARTESIAN_POINT ( 'NONE',  ( 35.90261398037149121, 14.17005867477686820, -8.593215200338315540 ) ) ;
#5307=VECTOR ( 'NONE', #35865, 1000.000000000000000 ) ;
#5311=ORIENTED_EDGE ( 'NONE', *, *, #18143, .T. ) ;
#5318=CARTESIAN_POINT ( 'NONE',  ( 54.86886719809545809, -45.79521720516596872, -17.39321520033831447 ) ) ;
#5319=ORIENTED_EDGE ( 'NONE', *, *, #18365, .F. ) ;
#5320=CARTESIAN_POINT ( 'NONE',  ( -2.326236797655081290, -6.982629615722759198, -7.609261158995283658 ) ) ;
#5337=EDGE_LOOP ( 'NONE', ( #2376, #16218, #13316, #13104 ) ) ;
#5339=CIRCLE ( 'NONE', #43231, 1.200000000000000178 ) ;
#5340=AXIS2_PLACEMENT_3D ( 'NONE', #17069, #38457, #38237 ) ;
#5354=CARTESIAN_POINT ( 'NONE',  ( 64.92272412734682518, -13.29087679925527254, -15.14070786268923285 ) ) ;
#5360=CARTESIAN_POINT ( 'NONE',  ( 67.43171844381110702, -0.1877862098377165168, -10.39321520033831625 ) ) ;
#5361=CARTESIAN_POINT ( 'NONE',  ( -2.501350073892645298, -7.035121566246528069, -19.26840662495741796 ) ) ;
#5375=DIRECTION ( 'NONE',  ( 0.000000000000000000, 0.000000000000000000, -1.000000000000000000 ) ) ;
#5378=CARTESIAN_POINT ( 'NONE',  ( -13.54490672864917045, -3.903797476764282681, -18.73945354926143736 ) ) ;
#5402=CARTESIAN_POINT ( 'NONE',  ( 62.10612082415807578, -3.658631476800715099, -7.496619392082022770 ) ) ;
#5474=CARTESIAN_POINT ( 'NONE',  ( 2.384484203314607420, -10.01861149699890063, -17.89321520033831447 ) ) ;
#5481=AXIS2_PLACEMENT_3D ( 'NONE', #3668, #41768, #27637 ) ;
#5501=ORIENTED_EDGE ( 'NONE', *, *, #32837, .T. ) ;
#5506=CARTESIAN_POINT ( 'NONE',  ( 65.62646388487864613, -15.45076938567549263, -16.39321520033831447 ) ) ;
#5527=EDGE_CURVE ( 'NONE', #11850, #27501, #44454, .T. ) ;
#5535=CARTESIAN_POINT ( 'NONE',  ( 64.28574602589941378, -2.825497480247340043, -18.75418257877172934 ) ) ;
#5538=CARTESIAN_POINT ( 'NONE',  ( -2.556913038227175416, -7.051771562855549291, -7.494178442794038553 ) ) ;
#5574=CIRCLE ( 'NONE', #38355, 1.199999999999999512 ) ;
#5575=CARTESIAN_POINT ( 'NONE',  ( 67.52182966331936598, -0.2245269270738840806, -10.39321520033831980 ) ) ;
#5593=CARTESIAN_POINT ( 'NONE',  ( -13.53629081928688649, -4.821193161180528541, -18.04471655251912665 ) ) ;
#5622=CARTESIAN_POINT ( 'NONE',  ( 66.99801899372408798, -0.07922336130813037447, -16.39321520033831447 ) ) ;
#5695=EDGE_CURVE ( 'NONE', #12923, #25838, #41270, .T. ) ;
#5699=ORIENTED_EDGE ( 'NONE', *, *, #41219, .F. ) ;
#5701=PLANE ( 'NONE',  #40124 ) ;
#5717=ORIENTED_EDGE ( 'NONE', *, *, #23481, .T. ) ;
#5742=DIRECTION ( 'NONE',  ( 0.000000000000000000, 0.000000000000000000, 1.000000000000000000 ) ) ;
#5754=CARTESIAN_POINT ( 'NONE',  ( 62.61854009670715726, -3.462514682154532952, -19.20073182371810461 ) ) ;
#5770=VERTEX_POINT ( 'NONE', #42150 ) ;
#5786=CARTESIAN_POINT ( 'NONE',  ( 66.58723489636778936, -20.14619392353143112, -19.39321520033831447 ) ) ;
#5790=AXIS2_PLACEMENT_3D ( 'NONE', #42439, #10315, #38108 ) ;
#5800=CARTESIAN_POINT ( 'NONE',  ( 67.42381492657879960, -0.1846631707194854588, -10.39321520033831625 ) ) ;
#5814=ADVANCED_FACE ( 'NONE', ( #38929 ), #185, .T. ) ;
#5819=CARTESIAN_POINT ( 'NONE',  ( -13.88591660730176436, -4.361019060476756692, -18.21192235134802928 ) ) ;
#5874=VERTEX_POINT ( 'NONE', #17969 ) ;
#5880=ORIENTED_EDGE ( 'NONE', *, *, #4755, .T. ) ;
#5906=CIRCLE ( 'NONE', #13116, 6.000000000000000888 ) ;
#5925=TOROIDAL_SURFACE ( 'NONE', #24873, 12.50000000000000000, 1.500000000000000000 ) ;
#5946=ORIENTED_EDGE ( 'NONE', *, *, #24219, .T. ) ;
#5961=CARTESIAN_POINT ( 'NONE',  ( 76.56645223742121686, 1.201885453592819397, -10.39321520033831625 ) ) ;
#5964=CIRCLE ( 'NONE', #30751, 4.999999999999997335 ) ;
#5970=VERTEX_POINT ( 'NONE', #32975 ) ;
#5973=CARTESIAN_POINT ( 'NONE',  ( 67.08264006073221708, -20.21382323020432992, -10.89321520033831447 ) ) ;
#5988=CIRCLE ( 'NONE', #27124, 1.200000000000000844 ) ;
#6004=CIRCLE ( 'NONE', #9666, 4.500000000000000888 ) ;
#6025=CARTESIAN_POINT ( 'NONE',  ( 60.53937939559665438, -4.256997083809236138, -8.893215200338314474 ) ) ;
#6029=CARTESIAN_POINT ( 'NONE',  ( 66.93334766501303079, -0.07218023934172421163, -10.39321520033831803 ) ) ;
#6035=FACE_BOUND ( 'NONE', #28332, .T. ) ;
#6043=CARTESIAN_POINT ( 'NONE',  ( 64.73784058450603140, -41.08681216603740438, -7.393215200338315363 ) ) ;
#6083=AXIS2_PLACEMENT_3D ( 'NONE', #32583, #39442, #4092 ) ;
#6085=EDGE_CURVE ( 'NONE', #25838, #873, #43269, .T. ) ;
#6114=EDGE_CURVE ( 'NONE', #41341, #2056, #43717, .T. ) ;
#6119=VERTEX_POINT ( 'NONE', #39396 ) ;
#6123=DIRECTION ( 'NONE',  ( -0.1352586133457944206, -0.9908103287288505534, 0.000000000000000000 ) ) ;
#6134=DIRECTION ( 'NONE',  ( 0.000000000000000000, 0.000000000000000000, -1.000000000000000000 ) ) ;
#6153=AXIS2_PLACEMENT_3D ( 'NONE', #35103, #3886, #24209 ) ;
#6197=FACE_BOUND ( 'NONE', #15997, .T. ) ;
#6224=AXIS2_PLACEMENT_3D ( 'NONE', #6025, #2605, #24055 ) ;
#6227=CARTESIAN_POINT ( 'NONE',  ( 59.62174278132244609, -14.86814543204979344, -18.19321520033831519 ) ) ;
#6256=CARTESIAN_POINT ( 'NONE',  ( 78.93021946355167984, -3.662536865724447921, -12.39321520033831447 ) ) ;
#6268=FACE_OUTER_BOUND ( 'NONE', #37286, .T. ) ;
#6269=CARTESIAN_POINT ( 'NONE',  ( -7.923679509334008664, -5.078949698970065540, -8.893215200338314474 ) ) ;
#6279=CARTESIAN_POINT ( 'NONE',  ( 0.04488520489200759078, -6.166763362545027327, -8.593215200338315540 ) ) ;
#6304=LINE ( 'NONE', #37762, #44953 ) ;
#6325=CARTESIAN_POINT ( 'NONE',  ( 75.14134903615895666, -42.50702760616825771, -10.89321520033831447 ) ) ;
#6332=DIRECTION ( 'NONE',  ( 0.000000000000000000, 0.000000000000000000, -1.000000000000000000 ) ) ;
#6341=DIRECTION ( 'NONE',  ( 0.000000000000000000, 0.000000000000000000, -1.000000000000000000 ) ) ;
#6360=EDGE_CURVE ( 'NONE', #15954, #32359, #26166, .T. ) ;
#6416=ORIENTED_EDGE ( 'NONE', *, *, #10709, .T. ) ;
#6437=EDGE_CURVE ( 'NONE', #12130, #41268, #23659, .T. ) ;
#6448=LINE ( 'NONE', #10319, #43137 ) ;
#6454=VERTEX_POINT ( 'NONE', #34779 ) ;
#6478=ADVANCED_FACE ( 'NONE', ( #20906 ), #37660, .T. ) ;
#6488=ADVANCED_FACE ( 'NONE', ( #42323 ), #28640, .T. ) ;
#6497=FACE_BOUND ( 'NONE', #35843, .T. ) ;
#6539=ADVANCED_FACE ( 'NONE', ( #4228 ), #3562, .T. ) ;
#6557=CYLINDRICAL_SURFACE ( 'NONE', #11118, 6.999999999999999112 ) ;
#6573=ORIENTED_EDGE ( 'NONE', *, *, #6437, .F. ) ;
#6578=VECTOR ( 'NONE', #25550, 1000.000000000000000 ) ;
#6585=ORIENTED_EDGE ( 'NONE', *, *, #12294, .F. ) ;
#6599=DIRECTION ( 'NONE',  ( 0.1352586133457953366, 0.9908103287288504424, 0.000000000000000000 ) ) ;
#6618=CARTESIAN_POINT ( 'NONE',  ( 60.06931813437629586, -14.72076136720887085, -19.39321520033831447 ) ) ;
#6624=VERTEX_POINT ( 'NONE', #21115 ) ;
#6646=CARTESIAN_POINT ( 'NONE',  ( 61.57437703972069443, -12.46983040987277214, -9.683387576578219580 ) ) ;
#6660=CARTESIAN_POINT ( 'NONE',  ( 42.57150613532612482, -13.18613447638990088, -19.39321520033831447 ) ) ;
#6667=ORIENTED_EDGE ( 'NONE', *, *, #29474, .T. ) ;
#6677=ORIENTED_EDGE ( 'NONE', *, *, #7215, .F. ) ;
#6698=EDGE_CURVE ( 'NONE', #12923, #23361, #1705, .T. ) ;
#6739=CIRCLE ( 'NONE', #22016, 1.499999999999999778 ) ;
#6741=LINE ( 'NONE', #6043, #25999 ) ;
#6748=LINE ( 'NONE', #12920, #39378 ) ;
#6765=VERTEX_POINT ( 'NONE', #43664 ) ;
#6777=DIRECTION ( 'NONE',  ( -0.9908103287288504424, 0.1352586133457950313, 0.000000000000000000 ) ) ;
#6791=VECTOR ( 'NONE', #553, 999.9999999999998863 ) ;
#6796=DIRECTION ( 'NONE',  ( 0.9063289528979890930, 0.4225728684367167087, 0.000000000000000000 ) ) ;
#6799=CARTESIAN_POINT ( 'NONE',  ( 0.04488520489200759078, -6.166763362545027327, -7.393215200338315363 ) ) ;
#6849=CIRCLE ( 'NONE', #32314, 4.499999999999994671 ) ;
#6852=ORIENTED_EDGE ( 'NONE', *, *, #4845, .T. ) ;
#6859=DIRECTION ( 'NONE',  ( 0.9908103287288506644, -0.1352586133457941986, 0.000000000000000000 ) ) ;
#6867=CARTESIAN_POINT ( 'NONE',  ( 63.13539060704677297, -12.63253393809564784, -10.30225669948812950 ) ) ;
#6879=CARTESIAN_POINT ( 'NONE',  ( 60.53937939559665438, -4.256997083809236138, -19.39321520033831447 ) ) ;
#6893=ORIENTED_EDGE ( 'NONE', *, *, #26511, .T. ) ;
#6899=DIRECTION ( 'NONE',  ( 0.1352586133457950590, 0.9908103287288504424, 0.000000000000000000 ) ) ;
#6941=EDGE_CURVE ( 'NONE', #33968, #6119, #13115, .T. ) ;
#6966=DIRECTION ( 'NONE',  ( 0.000000000000000000, 0.000000000000000000, -1.000000000000000000 ) ) ;
#6977=AXIS2_PLACEMENT_3D ( 'NONE', #28853, #42765, #5113 ) ;
#6982=ORIENTED_EDGE ( 'NONE', *, *, #40694, .F. ) ;
#6987=CARTESIAN_POINT ( 'NONE',  ( 71.31713442278440596, 2.423123680056959550, -10.60032198152486238 ) ) ;
#6995=DIRECTION ( 'NONE',  ( -0.4225728684367169308, 0.9063289528979889820, 0.000000000000000000 ) ) ;
#7043=CARTESIAN_POINT ( 'NONE',  ( 2.384484203314607420, -10.01861149699890063, -8.893215200338314474 ) ) ;
#7045=EDGE_CURVE ( 'NONE', #3982, #6624, #20226, .T. ) ;
#7050=DIRECTION ( 'NONE',  ( 0.3127730236694426513, -0.9498278979187093629, 0.000000000000000000 ) ) ;
#7071=ADVANCED_FACE ( 'NONE', ( #18605 ), #10045, .T. ) ;
#7082=EDGE_LOOP ( 'NONE', ( #23298, #34259, #11712, #33044 ) ) ;
#7083=CARTESIAN_POINT ( 'NONE',  ( 60.62063666025856179, -12.51771357505162285, -9.460505781647388091 ) ) ;
#7087=ORIENTED_EDGE ( 'NONE', *, *, #14827, .F. ) ;
#7088=ORIENTED_EDGE ( 'NONE', *, *, #9452, .T. ) ;
#7095=EDGE_CURVE ( 'NONE', #23894, #3183, #23624, .T. ) ;
#7096=CARTESIAN_POINT ( 'NONE',  ( 70.47992290675011873, 2.032776587329049978, -16.39321520033831447 ) ) ;
#7130=ORIENTED_EDGE ( 'NONE', *, *, #17537, .T. ) ;
#7149=CARTESIAN_POINT ( 'NONE',  ( 76.36356431740252049, -0.2843300395004543235, -14.39321520033831625 ) ) ;
#7157=ORIENTED_EDGE ( 'NONE', *, *, #20045, .F. ) ;
#7170=DIRECTION ( 'NONE',  ( 0.000000000000000000, 0.000000000000000000, 1.000000000000000000 ) ) ;
#7215=EDGE_CURVE ( 'NONE', #39449, #10182, #44249, .T. ) ;
#7244=( BOUNDED_CURVE ( )  B_SPLINE_CURVE ( 3, ( #1330, #880, #25290, #39418 ),
 .UNSPECIFIED., .F., .T. ) 
 B_SPLINE_CURVE_WITH_KNOTS ( ( 4, 4 ),
 ( 1.570796326794896558, 1.618943030528138038 ),
 .UNSPECIFIED. ) 
 CURVE ( )  GEOMETRIC_REPRESENTATION_ITEM ( )  RATIONAL_B_SPLINE_CURVE ( ( 1.000000000000000000, 0.9998068339056410680, 0.9998068339056410680, 1.000000000000000000 ) ) 
 REPRESENTATION_ITEM ( '' )  );
#7264=ORIENTED_EDGE ( 'NONE', *, *, #42709, .F. ) ;
#7272=ORIENTED_EDGE ( 'NONE', *, *, #22839, .F. ) ;
#7273=VECTOR ( 'NONE', #23552, 1000.000000000000000 ) ;
#7292=ORIENTED_EDGE ( 'NONE', *, *, #25608, .T. ) ;
#7307=CYLINDRICAL_SURFACE ( 'NONE', #6153, 1.200000000000000622 ) ;
#7309=DIRECTION ( 'NONE',  ( -0.9908103287288504424, 0.1352586133457950035, 0.000000000000000000 ) ) ;
#7343=AXIS2_PLACEMENT_3D ( 'NONE', #44879, #20702, #19618 ) ;
#7345=UNCERTAINTY_MEASURE_WITH_UNIT (LENGTH_MEASURE( 1.000000000000000082E-05 ), #8867, 'distance_accuracy_value', 'NONE');
#7410=CARTESIAN_POINT ( 'NONE',  ( 63.44904766417841557, -14.80807631840853134, -9.881358851643950558 ) ) ;
#7414=FACE_OUTER_BOUND ( 'NONE', #34440, .T. ) ;
#7415=DIRECTION ( 'NONE',  ( 0.9908103287288504424, -0.1352586133457950590, -0.000000000000000000 ) ) ;
#7420=DIRECTION ( 'NONE',  ( -1.000000000000000000, 0.000000000000000000, 0.000000000000000000 ) ) ;
#7442=LINE ( 'NONE', #7674, #1469 ) ;
#7493=DIRECTION ( 'NONE',  ( 0.1352586133457952255, 0.9908103287288504424, 0.000000000000000000 ) ) ;
#7500=CARTESIAN_POINT ( 'NONE',  ( 65.58061229095905276, -14.25342924908086673, -17.12691776711527325 ) ) ;
#7501=LINE ( 'NONE', #4756, #39197 ) ;
#7504=ORIENTED_EDGE ( 'NONE', *, *, #40126, .F. ) ;
#7515=DIRECTION ( 'NONE',  ( -1.000000000000000000, 0.000000000000000000, 0.000000000000000000 ) ) ;
#7546=CARTESIAN_POINT ( 'NONE',  ( 76.56645223742121686, 1.201885453592819397, -15.89321520033831447 ) ) ;
#7561=CARTESIAN_POINT ( 'NONE',  ( 63.13224612813448999, -13.41522658373937738, -18.64540057500950354 ) ) ;
#7591=DIRECTION ( 'NONE',  ( 0.000000000000000000, 0.000000000000000000, -1.000000000000000000 ) ) ;
#7606=ORIENTED_EDGE ( 'NONE', *, *, #1993, .T. ) ;
#7612=DIRECTION ( 'NONE',  ( -1.000000000000000000, 0.000000000000000000, 0.000000000000000000 ) ) ;
#7647=CARTESIAN_POINT ( 'NONE',  ( 60.61575878210037871, -12.54259051716152307, -17.30460924804371103 ) ) ;
#7648=CARTESIAN_POINT ( 'NONE',  ( -13.08016704199594393, -4.101600364181877900, -7.578546675885130313 ) ) ;
#7653=CARTESIAN_POINT ( 'NONE',  ( 63.51882515645636573, -14.83470500876697606, -9.935931153571182506 ) ) ;
#7674=CARTESIAN_POINT ( 'NONE',  ( 74.32979735608419958, -48.45188957854135481, -16.39321520033831447 ) ) ;
#7680=LINE ( 'NONE', #31625, #25437 ) ;
#7699=CARTESIAN_POINT ( 'NONE',  ( 64.68571552958836435, -2.672612419674116335, -8.182496787467194110 ) ) ;
#7728=CARTESIAN_POINT ( 'NONE',  ( 60.11760374155739584, -14.70486118635414385, -19.35686119223086266 ) ) ;
#7757=CARTESIAN_POINT ( 'NONE',  ( 35.90261398037149121, 14.17005867477686820, -7.393215200338315363 ) ) ;
#7779=ORIENTED_EDGE ( 'NONE', *, *, #29474, .F. ) ;
#7802=FACE_OUTER_BOUND ( 'NONE', #4773, .T. ) ;
#7806=EDGE_LOOP ( 'NONE', ( #39921, #42179, #16867, #17002 ) ) ;
#7812=CARTESIAN_POINT ( 'NONE',  ( 65.22670707961066228, -15.48412389236482412, -10.39321520033830737 ) ) ;
#7818=ORIENTED_EDGE ( 'NONE', *, *, #29071, .F. ) ;
#7854=CARTESIAN_POINT ( 'NONE',  ( 65.55689610126231059, -13.67296395165911704, -12.39321520033831447 ) ) ;
#7863=ORIENTED_EDGE ( 'NONE', *, *, #29071, .T. ) ;
#7881=CARTESIAN_POINT ( 'NONE',  ( -13.49829988753201881, -3.924578376762261733, -7.963090618125084674 ) ) ;
#7883=DIRECTION ( 'NONE',  ( 0.000000000000000000, 0.000000000000000000, 1.000000000000000000 ) ) ;
#7885=CARTESIAN_POINT ( 'NONE',  ( 64.20808384960839987, -15.18003272038575524, -10.58763554360807646 ) ) ;
#7890=ORIENTED_EDGE ( 'NONE', *, *, #16982, .T. ) ;
#7911=CARTESIAN_POINT ( 'NONE',  ( 61.77615262425602793, -2.025327440714448812, -17.89321520033831447 ) ) ;
#7922=ORIENTED_EDGE ( 'NONE', *, *, #4258, .T. ) ;
#7927=CARTESIAN_POINT ( 'NONE',  ( -12.52970885032985748, -4.316676466568440063, -7.393215200338314474 ) ) ;
#7942=VERTEX_POINT ( 'NONE', #16493 ) ;
#7945=CARTESIAN_POINT ( 'NONE',  ( 69.69189222815028018, -41.76310523276638520, -16.39321520033831447 ) ) ;
#7955=CARTESIAN_POINT ( 'NONE',  ( 59.75121349346654398, -13.58877957849836093, -19.38162691376808411 ) ) ;
#7968=B_SPLINE_CURVE_WITH_KNOTS ( 'NONE', 3,
 ( #27935, #21076, #28826, #38609, #39305, #8076, #21977, #554, #34953, #3739, #14239, #42066, #10823, #24721 ),
 .UNSPECIFIED., .F., .F.,
 ( 4, 2, 2, 2, 2, 2, 4 ),
 ( 6.938893903907228378E-18, 0.001308732638115193449, 0.001963098957172786704, 0.002617465276230379959, 0.003271831595287972780, 0.003926197914345566468, 0.005234930552460722621 ),
 .UNSPECIFIED. ) ;
#7969=LINE ( 'NONE', #671, #39773 ) ;
#7975=CARTESIAN_POINT ( 'NONE',  ( 65.70844687201810075, -0.1919082892013201924, -16.07106790048558054 ) ) ;
#7976=EDGE_LOOP ( 'NONE', ( #20057, #10055, #41376, #11804 ) ) ;
#7990=FACE_OUTER_BOUND ( 'NONE', #2760, .T. ) ;
#7999=DIRECTION ( 'NONE',  ( -0.9908103287288504424, 0.1352586133457951423, 0.000000000000000000 ) ) ;
#8005=ORIENTED_EDGE ( 'NONE', *, *, #40657, .T. ) ;
#8040=ORIENTED_EDGE ( 'NONE', *, *, #7045, .T. ) ;
#8057=ORIENTED_EDGE ( 'NONE', *, *, #17794, .F. ) ;
#8060=FACE_OUTER_BOUND ( 'NONE', #5337, .T. ) ;
#8062=DIRECTION ( 'NONE',  ( 0.000000000000000000, 0.000000000000000000, 1.000000000000000000 ) ) ;
#8065=ORIENTED_EDGE ( 'NONE', *, *, #31406, .T. ) ;
#8076=CARTESIAN_POINT ( 'NONE',  ( 62.16677121967738628, -14.49431128105000610, -17.68377221324302795 ) ) ;
#8086=CARTESIAN_POINT ( 'NONE',  ( 31.33087284928346605, -19.31933043625825874, -18.19321520033831519 ) ) ;
#8101=AXIS2_PLACEMENT_3D ( 'NONE', #19558, #30045, #43961 ) ;
#8117=CARTESIAN_POINT ( 'NONE',  ( 62.28506180665693392, -13.31920281343605339, -7.834338051647534940 ) ) ;
#8121=EDGE_LOOP ( 'NONE', ( #15938, #41978 ) ) ;
#8158=ORIENTED_EDGE ( 'NONE', *, *, #35297, .F. ) ;
#8160=CARTESIAN_POINT ( 'NONE',  ( -13.88569750198904806, -4.361307444782807075, -8.573647932902863644 ) ) ;
#8163=CARTESIAN_POINT ( 'NONE',  ( 66.82983677891284913, -0.05992252863833068266, -16.39321520033831803 ) ) ;
#8219=DIRECTION ( 'NONE',  ( 0.000000000000000000, 0.000000000000000000, 1.000000000000000000 ) ) ;
#8235=ORIENTED_EDGE ( 'NONE', *, *, #43431, .F. ) ;
#8241=CARTESIAN_POINT ( 'NONE',  ( -13.08039557466221048, -4.101515749868387850, -19.20787527460400312 ) ) ;
#8265=ORIENTED_EDGE ( 'NONE', *, *, #32837, .F. ) ;
#8272=AXIS2_PLACEMENT_3D ( 'NONE', #26139, #42178, #14356 ) ;
#8276=CIRCLE ( 'NONE', #33750, 4.999999999999999112 ) ;
#8296=CARTESIAN_POINT ( 'NONE',  ( -11.17889843615491685, -5.940389178047622565, -19.39321520033831447 ) ) ;
#8297=DIRECTION ( 'NONE',  ( -0.1352586133457950590, -0.9908103287288504424, 0.000000000000000000 ) ) ;
#8301=DIRECTION ( 'NONE',  ( -0.1352586133457950590, -0.9908103287288504424, 0.000000000000000000 ) ) ;
#8332=CARTESIAN_POINT ( 'NONE',  ( 64.83175385985305184, -13.24295385337449460, -15.23335304249422428 ) ) ;
#8338=CARTESIAN_POINT ( 'NONE',  ( 64.04456645099679690, -15.08556008563613204, -10.41505815062060236 ) ) ;
#8360=CARTESIAN_POINT ( 'NONE',  ( 60.45894907855897316, -4.846173528048923096, -9.393215200338314474 ) ) ;
#8376=EDGE_LOOP ( 'NONE', ( #43299, #29528, #12858, #7272, #30359, #13405 ) ) ;
#8400=AXIS2_PLACEMENT_3D ( 'NONE', #31521, #28119, #42026 ) ;
#8423=( NAMED_UNIT ( * ) SI_UNIT ( $, .STERADIAN. ) SOLID_ANGLE_UNIT ( ) );
#8433=AXIS2_PLACEMENT_3D ( 'NONE', #25208, #34980, #4665 ) ;
#8436=ORIENTED_EDGE ( 'NONE', *, *, #21102, .F. ) ;
#8446=CARTESIAN_POINT ( 'NONE',  ( 3.060777270043529619, -5.064559853354640317, -7.393215200338315363 ) ) ;
#8472=DIRECTION ( 'NONE',  ( -0.4225728684367210941, 0.9063289528979869836, 0.000000000000000000 ) ) ;
#8493=EDGE_CURVE ( 'NONE', #18952, #20112, #18450, .T. ) ;
#8523=CIRCLE ( 'NONE', #33239, 1.200000000000000178 ) ;
#8541=VERTEX_POINT ( 'NONE', #34839 ) ;
#8552=CYLINDRICAL_SURFACE ( 'NONE', #38978, 1.499999999999998002 ) ;
#8555=CARTESIAN_POINT ( 'NONE',  ( 65.55689610126231059, -13.67296395165911704, -14.39321520033831625 ) ) ;
#8559=VECTOR ( 'NONE', #1263, 1000.000000000000000 ) ;
#8564=CARTESIAN_POINT ( 'NONE',  ( 62.83933201006751545, -13.37155033267121951, -8.024690356892984155 ) ) ;
#8632=CARTESIAN_POINT ( 'NONE',  ( 59.75121349346655109, -13.58877957849837692, -7.404803486908546617 ) ) ;
#8724=DIRECTION ( 'NONE',  ( 0.000000000000000000, 0.000000000000000000, 1.000000000000000000 ) ) ;
#8739=DIRECTION ( 'NONE',  ( 0.000000000000000000, 0.000000000000000000, 1.000000000000000000 ) ) ;
#8742=CARTESIAN_POINT ( 'NONE',  ( -1.803662125172398545, -6.825544624776664904, -8.166198927921115569 ) ) ;
#8749=VECTOR ( 'NONE', #30706, 1000.000000000000000 ) ;
#8782=CARTESIAN_POINT ( 'NONE',  ( 66.90558936096920206, -0.06963689119154935214, -10.39321520033831803 ) ) ;
#8787=EDGE_LOOP ( 'NONE', ( #34111, #19882, #40972, #9487 ) ) ;
#8801=CARTESIAN_POINT ( 'NONE',  ( -12.52947101616301673, -4.316762297166332196, -19.39321520033831803 ) ) ;
#8828=DIRECTION ( 'NONE',  ( 0.000000000000000000, 0.000000000000000000, 1.000000000000000000 ) ) ;
#8830=CARTESIAN_POINT ( 'NONE',  ( 66.16515534780279495, -0.1171416179790299994, -16.39321520033831803 ) ) ;
#8845=CARTESIAN_POINT ( 'NONE',  ( -7.923679509334008664, -5.078949698970065540, -8.893215200338314474 ) ) ;
#8860=EDGE_CURVE ( 'NONE', #35546, #5970, #28275, .T. ) ;
#8867=( LENGTH_UNIT ( ) NAMED_UNIT ( * ) SI_UNIT ( .MILLI., .METRE. ) );
#8903=ORIENTED_EDGE ( 'NONE', *, *, #35051, .F. ) ;
#8928=ORIENTED_EDGE ( 'NONE', *, *, #41494, .F. ) ;
#8947=EDGE_CURVE ( 'NONE', #33232, #13961, #7501, .T. ) ;
#8958=EDGE_LOOP ( 'NONE', ( #31828, #3939, #14652, #11833 ) ) ;
#8973=DIRECTION ( 'NONE',  ( 0.000000000000000000, 0.000000000000000000, 1.000000000000000000 ) ) ;
#8982=DIRECTION ( 'NONE',  ( -0.1352586133457981954, -0.9908103287288499983, 0.000000000000000000 ) ) ;
#8991=ORIENTED_EDGE ( 'NONE', *, *, #33478, .F. ) ;
#9012=CARTESIAN_POINT ( 'NONE',  ( 67.08264006073221708, -20.21382323020432992, -10.89321520033831447 ) ) ;
#9021=VERTEX_POINT ( 'NONE', #2232 ) ;
#9029=CARTESIAN_POINT ( 'NONE',  ( 68.56885555382550024, -20.41671115022304406, -12.39321520033831447 ) ) ;
#9031=CARTESIAN_POINT ( 'NONE',  ( -13.38014282662990162, -5.026713647828855436, -8.593215200338319093 ) ) ;
#9040=DIRECTION ( 'NONE',  ( 0.7962509850245457210, 0.6049664196031383501, 0.000000000000000000 ) ) ;
#9041=EDGE_LOOP ( 'NONE', ( #32417, #3373, #20530, #37592 ) ) ;
#9053=ORIENTED_EDGE ( 'NONE', *, *, #6698, .T. ) ;
#9060=ADVANCED_FACE ( 'NONE', ( #15479 ), #43296, .T. ) ;
#9061=CARTESIAN_POINT ( 'NONE',  ( 67.26988314049960138, -0.1294138187462419431, -16.39321520033831447 ) ) ;
#9071=VERTEX_POINT ( 'NONE', #12519 ) ;
#9086=ORIENTED_EDGE ( 'NONE', *, *, #44338, .F. ) ;
#9107=DIRECTION ( 'NONE',  ( 0.000000000000000000, 0.000000000000000000, -1.000000000000000000 ) ) ;
#9181=ORIENTED_EDGE ( 'NONE', *, *, #10964, .F. ) ;
#9182=VECTOR ( 'NONE', #42713, 1000.000000000000000 ) ;
#9202=CARTESIAN_POINT ( 'NONE',  ( -2.533732661084656002, -7.044826992859106518, -7.503826880137411059 ) ) ;
#9240=CARTESIAN_POINT ( 'NONE',  ( 65.10287265247758626, -0.4742552606671335269, -10.39321520033831625 ) ) ;
#9245=VERTEX_POINT ( 'NONE', #37107 ) ;
#9256=DIRECTION ( 'NONE',  ( -0.9908103287288505534, 0.1352586133457950313, 0.000000000000000000 ) ) ;
#9259=CARTESIAN_POINT ( 'NONE',  ( -13.49558570875300134, -4.874768836305437780, -18.10912819220449421 ) ) ;
#9275=ORIENTED_EDGE ( 'NONE', *, *, #17740, .T. ) ;
#9289=LINE ( 'NONE', #13166, #36909 ) ;
#9302=DIRECTION ( 'NONE',  ( -0.9908103287288504424, 0.1352586133457950590, 0.000000000000000000 ) ) ;
#9310=DIRECTION ( 'NONE',  ( -0.9063289528979890930, -0.4225728684367167087, 0.000000000000000000 ) ) ;
#9334=DIRECTION ( 'NONE',  ( -0.9908103287288504424, 0.1352586133457951423, 0.000000000000000000 ) ) ;
#9336=ORIENTED_EDGE ( 'NONE', *, *, #1314, .F. ) ;
#9360=CARTESIAN_POINT ( 'NONE',  ( -7.917624645353499524, -12.21642755857638818, -18.19321520033831519 ) ) ;
#9411=ORIENTED_EDGE ( 'NONE', *, *, #2440, .F. ) ;
#9416=CARTESIAN_POINT ( 'NONE',  ( 63.37404594698951854, -3.173945195454633605, -19.03816892419136764 ) ) ;
#9439=EDGE_CURVE ( 'NONE', #873, #23361, #44212, .T. ) ;
#9445=DIRECTION ( 'NONE',  ( 0.9908103287288495542, -0.1352586133458027196, 0.000000000000000000 ) ) ;
#9448=CARTESIAN_POINT ( 'NONE',  ( 59.62174278132245320, -14.86814543204979344, -7.393215200338313586 ) ) ;
#9452=EDGE_CURVE ( 'NONE', #26347, #32179, #14447, .T. ) ;
#9456=EDGE_CURVE ( 'NONE', #23894, #3386, #7680, .T. ) ;
#9478=CARTESIAN_POINT ( 'NONE',  ( 59.69399050597296252, -13.58096788970641811, -8.603412892520118760 ) ) ;
#9487=ORIENTED_EDGE ( 'NONE', *, *, #12819, .T. ) ;
#9504=ORIENTED_EDGE ( 'NONE', *, *, #37847, .F. ) ;
#9542=ORIENTED_EDGE ( 'NONE', *, *, #42709, .T. ) ;
#9549=FACE_OUTER_BOUND ( 'NONE', #30433, .T. ) ;
#9553=AXIS2_PLACEMENT_3D ( 'NONE', #29824, #36872, #26406 ) ;
#9605=CARTESIAN_POINT ( 'NONE',  ( 61.41452964936473791, -3.848961180437260321, -19.39321520033831447 ) ) ;
#9653=ORIENTED_EDGE ( 'NONE', *, *, #14201, .F. ) ;
#9654=CARTESIAN_POINT ( 'NONE',  ( -3.075987277002964593, -7.207016596002466358, -7.393215200338315363 ) ) ;
#9666=AXIS2_PLACEMENT_3D ( 'NONE', #34604, #3389, #44905 ) ;
#9680=CARTESIAN_POINT ( 'NONE',  ( -7.923679509334008664, -5.078949698970065540, -17.89321520033831447 ) ) ;
#9694=CARTESIAN_POINT ( 'NONE',  ( -2.989246886974374462, -7.181049323750285929, -19.39371206063207254 ) ) ;
#9695=FACE_OUTER_BOUND ( 'NONE', #4977, .T. ) ;
#9708=DIRECTION ( 'NONE',  ( 0.000000000000000000, 0.000000000000000000, 1.000000000000000000 ) ) ;
#9793=EDGE_CURVE ( 'NONE', #16955, #27202, #18885, .T. ) ;
#9807=VECTOR ( 'NONE', #1415, 1000.000000000000000 ) ;
#9816=ORIENTED_EDGE ( 'NONE', *, *, #3869, .F. ) ;
#9825=DIRECTION ( 'NONE',  ( 0.000000000000000000, 0.000000000000000000, 1.000000000000000000 ) ) ;
#9859=PLANE ( 'NONE',  #349 ) ;
#9950=DIRECTION ( 'NONE',  ( 0.6049664196031386831, -0.7962509850245457210, 0.000000000000000000 ) ) ;
#9953=AXIS2_PLACEMENT_3D ( 'NONE', #35771, #24851, #32356 ) ;
#9967=EDGE_LOOP ( 'NONE', ( #39098, #40475, #39123, #40858 ) ) ;
#9978=DIRECTION ( 'NONE',  ( 0.6049664196031393493, -0.7962509850245451659, -0.000000000000000000 ) ) ;
#9988=EDGE_CURVE ( 'NONE', #43799, #23752, #10858, .T. ) ;
#9996=FACE_OUTER_BOUND ( 'NONE', #14627, .T. ) ;
#9999=ORIENTED_EDGE ( 'NONE', *, *, #19187, .T. ) ;
#10008=ORIENTED_EDGE ( 'NONE', *, *, #19286, .F. ) ;
#10020=CARTESIAN_POINT ( 'NONE',  ( 77.44400397045842510, -3.459648945705700473, -12.39321520033831447 ) ) ;
#10024=LINE ( 'NONE', #30979, #2355 ) ;
#10030=CARTESIAN_POINT ( 'NONE',  ( 2.384484203314607420, -10.01861149699890063, -17.89321520033831447 ) ) ;
#10045=TOROIDAL_SURFACE ( 'NONE', #35489, 5.500000000000000000, 0.5000000000000000000 ) ;
#10055=ORIENTED_EDGE ( 'NONE', *, *, #17740, .F. ) ;
#10066=VECTOR ( 'NONE', #27308, 1000.000000000000000 ) ;
#10079=CARTESIAN_POINT ( 'NONE',  ( 61.78823460971035786, -12.47025219434260457, -9.744219563062513245 ) ) ;
#10084=VERTEX_POINT ( 'NONE', #11446 ) ;
#10091=CYLINDRICAL_SURFACE ( 'NONE', #41545, 0.5000000000000035527 ) ;
#10110=CARTESIAN_POINT ( 'NONE',  ( 59.77099224207091765, -14.81899841792058048, -18.19321520033777162 ) ) ;
#10114=DIRECTION ( 'NONE',  ( -0.9908103287288504424, 0.1352586133457950590, 0.000000000000000000 ) ) ;
#10133=CARTESIAN_POINT ( 'NONE',  ( -13.78505786849281911, -3.796669023460694792, -8.893215200338314474 ) ) ;
#10167=PLANE ( 'NONE',  #15280 ) ;
#10173=B_SPLINE_CURVE_WITH_KNOTS ( 'NONE', 3,
 ( #28938, #43294, #12064, #42623, #39649, #32566, #35760, #38959 ),
 .UNSPECIFIED., .F., .F.,
 ( 4, 2, 2, 4 ),
 ( 0.000000000000000000, 0.0001409761270367683526, 0.0002819522540735367052, 0.0005639045081470742777 ),
 .UNSPECIFIED. ) ;
#10182=VERTEX_POINT ( 'NONE', #36264 ) ;
#10207=CARTESIAN_POINT ( 'NONE',  ( 68.56885555382550024, -20.41671115022304406, -14.39321520033831625 ) ) ;
#10269=CARTESIAN_POINT ( 'NONE',  ( 2.181596283295915484, -11.50482699009217669, -19.39321520033831447 ) ) ;
#10274=EDGE_CURVE ( 'NONE', #27202, #16290, #38187, .T. ) ;
#10292=ORIENTED_EDGE ( 'NONE', *, *, #33887, .F. ) ;
#10293=CIRCLE ( 'NONE', #1446, 1.499999999999998002 ) ;
#10308=CARTESIAN_POINT ( 'NONE',  ( 59.36680634945873436, -12.84644995903807541, -9.393215200338314474 ) ) ;
#10315=DIRECTION ( 'NONE',  ( 0.000000000000000000, 0.000000000000000000, 1.000000000000000000 ) ) ;
#10319=CARTESIAN_POINT ( 'NONE',  ( 72.51188087854242781, -21.10583385764521225, -7.393215200338315363 ) ) ;
#10349=ORIENTED_EDGE ( 'NONE', *, *, #26741, .T. ) ;
#10353=ORIENTED_EDGE ( 'NONE', *, *, #39824, .T. ) ;
#10357=PRODUCT_DEFINITION ( 'UNKNOWN', '', #35863, #15095 ) ;
#10371=CIRCLE ( 'NONE', #24206, 4.999999999999998224 ) ;
#10419=CARTESIAN_POINT ( 'NONE',  ( 62.84522113422936940, -12.57561100918773178, -16.63017181072184769 ) ) ;
#10428=LINE ( 'NONE', #10648, #33316 ) ;
#10441=B_SPLINE_CURVE_WITH_KNOTS ( 'NONE', 3,
 ( #11555, #9031, #29999, #22703, #36151, #32507, #25463, #43466 ),
 .UNSPECIFIED., .F., .F.,
 ( 4, 2, 2, 4 ),
 ( 0.000000000000000000, 0.0002795070773440827094, 0.0004192606160161267475, 0.0005590141546881708398 ),
 .UNSPECIFIED. ) ;
#10473=CYLINDRICAL_SURFACE ( 'NONE', #27348, 1.199999999999998623 ) ;
#10475=DIRECTION ( 'NONE',  ( -0.9908103287288504424, 0.1352586133457950313, 0.000000000000000000 ) ) ;
#10490=ORIENTED_EDGE ( 'NONE', *, *, #32531, .F. ) ;
#10514=CARTESIAN_POINT ( 'NONE',  ( 62.35708470706295969, -12.50172482834998178, -9.937585253968853394 ) ) ;
#10524=CARTESIAN_POINT ( 'NONE',  ( 75.95778847736514194, -3.256761025687008537, -10.39321520033831625 ) ) ;
#10525=ADVANCED_FACE ( 'NONE', ( #35884 ), #39324, .T. ) ;
#10566=ORIENTED_EDGE ( 'NONE', *, *, #13240, .F. ) ;
#10572=CYLINDRICAL_SURFACE ( 'NONE', #15773, 6.000000000000005329 ) ;
#10610=CARTESIAN_POINT ( 'NONE',  ( 71.31713442278437753, 2.423123680056944007, -19.39321520033831447 ) ) ;
#10620=AXIS2_PLACEMENT_3D ( 'NONE', #31366, #32035, #14052 ) ;
#10630=CARTESIAN_POINT ( 'NONE',  ( 64.66985656418735573, -0.6761475757289143740, -10.04201475645285591 ) ) ;
#10637=CARTESIAN_POINT ( 'NONE',  ( 61.49539530949622446, -12.46540452739392890, -17.12947030793335657 ) ) ;
#10638=ADVANCED_FACE ( 'NONE', ( #24001 ), #26736, .F. ) ;
#10643=DIRECTION ( 'NONE',  ( -0.9063289528979890930, -0.4225728684367167087, -3.263703555153020391E-15 ) ) ;
#10648=CARTESIAN_POINT ( 'NONE',  ( 74.64594387179452895, -42.43939829949535181, -7.393215200338315363 ) ) ;
#10663=EDGE_CURVE ( 'NONE', #9021, #34939, #45132, .T. ) ;
#10678=CIRCLE ( 'NONE', #36133, 1.499999999999999556 ) ;
#10685=DIRECTION ( 'NONE',  ( 0.1352586133457950590, 0.9908103287288504424, 0.000000000000000000 ) ) ;
#10709=EDGE_CURVE ( 'NONE', #32359, #23226, #35634, .T. ) ;
#10716=CARTESIAN_POINT ( 'NONE',  ( 64.51289607492564926, -15.37840541894191126, -15.84259706628786724 ) ) ;
#10727=DIRECTION ( 'NONE',  ( 1.000000000000000000, 0.000000000000000000, 0.000000000000000000 ) ) ;
#10729=DIRECTION ( 'NONE',  ( 0.1352586133457950590, 0.9908103287288504424, 0.000000000000000000 ) ) ;
#10731=DIRECTION ( 'NONE',  ( 0.000000000000000000, 0.000000000000000000, -1.000000000000000000 ) ) ;
#10748=AXIS2_PLACEMENT_3D ( 'NONE', #13795, #31110, #44815 ) ;
#10770=CARTESIAN_POINT ( 'NONE',  ( 76.36356431740252049, -0.2843300395004543235, -19.39321520033831447 ) ) ;
#10823=CARTESIAN_POINT ( 'NONE',  ( 64.21381391892587942, -15.17632890891008479, -16.20372347372216026 ) ) ;
#10858=CIRCLE ( 'NONE', #42168, 0.5000000000000043299 ) ;
#10913=EDGE_CURVE ( 'NONE', #24167, #4486, #478, .T. ) ;
#10928=AXIS2_PLACEMENT_3D ( 'NONE', #27548, #6341, #34798 ) ;
#10935=CARTESIAN_POINT ( 'NONE',  ( 64.06702676307045863, -13.62987338852582653, -18.19193609654278276 ) ) ;
#10949=CARTESIAN_POINT ( 'NONE',  ( 31.16203868753470019, 11.28474725185576055, -19.39321520033831447 ) ) ;
#10964=EDGE_CURVE ( 'NONE', #35887, #5874, #44123, .T. ) ;
#10977=ORIENTED_EDGE ( 'NONE', *, *, #8493, .T. ) ;
#10980=CARTESIAN_POINT ( 'NONE',  ( 69.69189222815028018, -41.76310523276638520, -10.39321520033831625 ) ) ;
#10988=ORIENTED_EDGE ( 'NONE', *, *, #6360, .F. ) ;
#10993=( BOUNDED_SURFACE ( )  B_SPLINE_SURFACE ( 3, 2, ( 
 ( #44795, #9448, #24268 ),
 ( #41602, #31093, #30651 ),
 ( #34284, #33827, #38156 ),
 ( #24045, #2598, #23362 ) ),
 .UNSPECIFIED., .F., .F., .F. ) 
 B_SPLINE_SURFACE_WITH_KNOTS ( ( 4, 4 ),
 ( 3, 3 ),
 ( 1.570796326794896558, 1.618943030528137816 ),
 ( 0.000000000000000000, 1.000000000000000000 ),
 .UNSPECIFIED. ) 
 GEOMETRIC_REPRESENTATION_ITEM ( )  RATIONAL_B_SPLINE_SURFACE ( (
 ( 1.000000000000000000, 0.7071067811865475727, 1.000000000000000000),
 ( 1.000000000000000000, 0.7095941637304925553, 1.000000000000000000),
 ( 1.000000000000000000, 0.7120684114869151315, 1.000000000000000000),
 ( 1.000000000000000000, 0.7145271066604789167, 1.000000000000000000) ) ) 
 REPRESENTATION_ITEM ( '' )  SURFACE ( )  );
#10995=CARTESIAN_POINT ( 'NONE',  ( -13.23547271986589990, -4.036892331970093117, -19.09970410335115787 ) ) ;
#11018=VERTEX_POINT ( 'NONE', #1591 ) ;
#11025=EDGE_LOOP ( 'NONE', ( #1417, #7779, #10988, #44727 ) ) ;
#11026=CARTESIAN_POINT ( 'NONE',  ( 75.95778847736514194, -3.256761025687008537, -7.147228641687434880 ) ) ;
#11039=ORIENTED_EDGE ( 'NONE', *, *, #39491, .T. ) ;
#11053=DIRECTION ( 'NONE',  ( -0.9908103287288504424, 0.1352586133457951423, 0.000000000000000000 ) ) ;
#11072=CARTESIAN_POINT ( 'NONE',  ( 61.76166819791257012, -14.46743153019240147, -8.940005687461745509 ) ) ;
#11082=CARTESIAN_POINT ( 'NONE',  ( -13.78505786849281911, -3.796669023460695680, -8.693443890614471314 ) ) ;
#11093=EDGE_LOOP ( 'NONE', ( #24112, #23835, #30626, #11180 ) ) ;
#11118=AXIS2_PLACEMENT_3D ( 'NONE', #44874, #6332, #13630 ) ;
#11124=CIRCLE ( 'NONE', #18380, 12.50000000000000178 ) ;
#11133=CARTESIAN_POINT ( 'NONE',  ( 64.70242381814703947, -2.666228601359576622, -8.189135705538296506 ) ) ;
#11140=AXIS2_PLACEMENT_3D ( 'NONE', #17078, #6123, #20042 ) ;
#11150=VERTEX_POINT ( 'NONE', #27870 ) ;
#11158=ORIENTED_EDGE ( 'NONE', *, *, #38394, .F. ) ;
#11161=CARTESIAN_POINT ( 'NONE',  ( 59.41476255453773803, -13.68180535374018092, -19.39321520033831803 ) ) ;
#11162=CARTESIAN_POINT ( 'NONE',  ( 64.18180727272476815, -15.10249645379742667, -18.01844049509142920 ) ) ;
#11180=ORIENTED_EDGE ( 'NONE', *, *, #18143, .F. ) ;
#11184=CARTESIAN_POINT ( 'NONE',  ( 59.90552009294157898, -2.897503654462289191, -17.89321520033831447 ) ) ;
#11221=CARTESIAN_POINT ( 'NONE',  ( -13.60484295501412433, -3.877462935949435252, -18.65581272914820588 ) ) ;
#11249=ORIENTED_EDGE ( 'NONE', *, *, #18431, .T. ) ;
#11257=CARTESIAN_POINT ( 'NONE',  ( -13.56828337869050927, -4.779084862086334873, -8.893215200338314474 ) ) ;
#11271=LINE ( 'NONE', #8296, #6791 ) ;
#11273=DIRECTION ( 'NONE',  ( -0.1352586133457950590, -0.9908103287288504424, 0.000000000000000000 ) ) ;
#11279=CARTESIAN_POINT ( 'NONE',  ( 65.37216319521120056, -13.55122928640068913, -12.15172136135480230 ) ) ;
#11287=ORIENTED_EDGE ( 'NONE', *, *, #4454, .F. ) ;
#11310=CARTESIAN_POINT ( 'NONE',  ( 64.39952598912073256, -15.22865974175013015, -8.907941765600535078 ) ) ;
#11323=CIRCLE ( 'NONE', #11353, 25.00000000000000355 ) ;
#11353=AXIS2_PLACEMENT_3D ( 'NONE', #42655, #25332, #18257 ) ;
#11364=EDGE_CURVE ( 'NONE', #11150, #16401, #20080, .T. ) ;
#11399=COLOUR_RGB ( '',0.7921568627450980005, 0.8196078431372548767, 0.9333333333333333481 ) ;
#11400=CARTESIAN_POINT ( 'NONE',  ( 69.69189222815028018, -41.76310523276638520, -7.393215200338315363 ) ) ;
#11401=CARTESIAN_POINT ( 'NONE',  ( 59.90552009294157898, -2.897503654462289191, -8.893215200338314474 ) ) ;
#11409=CARTESIAN_POINT ( 'NONE',  ( 65.53668513659742700, -0.2719916286899254909, -18.52721583069677180 ) ) ;
#11410=VERTEX_POINT ( 'NONE', #44257 ) ;
#11446=CARTESIAN_POINT ( 'NONE',  ( 31.16856251326850824, -20.50830283073288385, -8.593215200338315540 ) ) ;
#11448=CARTESIAN_POINT ( 'NONE',  ( 59.75121349346655109, -13.58877957849837692, -19.38162691376808411 ) ) ;
#11462=ORIENTED_EDGE ( 'NONE', *, *, #16709, .F. ) ;
#11468=DIRECTION ( 'NONE',  ( -0.9063289528979890930, -0.4225728684367167087, 0.000000000000000000 ) ) ;
#11520=TOROIDAL_SURFACE ( 'NONE', #36963, 5.500000000000000000, 0.5000000000000000000 ) ;
#11535=DIRECTION ( 'NONE',  ( 0.000000000000000000, 0.000000000000000000, -1.000000000000000000 ) ) ;
#11537=LINE ( 'NONE', #31819, #2749 ) ;
#11540=CARTESIAN_POINT ( 'NONE',  ( 66.12481753886987690, -14.57890275351189402, -10.17775628694920087 ) ) ;
#11555=CARTESIAN_POINT ( 'NONE',  ( -13.32377113153209791, -5.100909530930220370, -8.593215200338315540 ) ) ;
#11580=ORIENTED_EDGE ( 'NONE', *, *, #21934, .F. ) ;
#11582=CARTESIAN_POINT ( 'NONE',  ( 64.66798275244620697, -2.679388005794879568, -8.175474704283455907 ) ) ;
#11597=ORIENTED_EDGE ( 'NONE', *, *, #44692, .T. ) ;
#11608=CARTESIAN_POINT ( 'NONE',  ( 63.13926143489126730, -14.69785589905574241, -17.13608958866837639 ) ) ;
#11616=( NAMED_UNIT ( * ) PLANE_ANGLE_UNIT ( ) SI_UNIT ( $, .RADIAN. ) );
#11619=CARTESIAN_POINT ( 'NONE',  ( 61.77615262425602793, -2.025327440714448812, -8.893215200338310922 ) ) ;
#11624=CARTESIAN_POINT ( 'NONE',  ( 68.27538871269578635, -1.300937240615723800, -16.26478957841321460 ) ) ;
#11625=ORIENTED_EDGE ( 'NONE', *, *, #12309, .F. ) ;
#11638=LINE ( 'NONE', #24872, #6578 ) ;
#11639=VECTOR ( 'NONE', #7170, 1000.000000000000000 ) ;
#11650=ORIENTED_EDGE ( 'NONE', *, *, #1993, .F. ) ;
#11661=DIRECTION ( 'NONE',  ( -0.1352586133457954198, -0.9908103287288503314, 0.000000000000000000 ) ) ;
#11664=CARTESIAN_POINT ( 'NONE',  ( 65.91876108126253087, -14.44801200876193370, -16.81557847985648735 ) ) ;
#11669=ORIENTED_EDGE ( 'NONE', *, *, #12672, .T. ) ;
#11703=DIRECTION ( 'NONE',  ( 0.9908103287288505534, -0.1352586133457950590, 0.000000000000000000 ) ) ;
#11707=DIRECTION ( 'NONE',  ( 0.000000000000000000, 0.000000000000000000, 1.000000000000000000 ) ) ;
#11712=ORIENTED_EDGE ( 'NONE', *, *, #31701, .F. ) ;
#11722=VERTEX_POINT ( 'NONE', #8632 ) ;
#11729=DIRECTION ( 'NONE',  ( 0.9908103287288504424, -0.1352586133457950313, 0.000000000000000000 ) ) ;
#11749=FACE_OUTER_BOUND ( 'NONE', #40486, .T. ) ;
#11754=CARTESIAN_POINT ( 'NONE',  ( 64.98755411081816646, -13.32594127658043170, -15.07288939246319970 ) ) ;
#11759=CARTESIAN_POINT ( 'NONE',  ( -1.637506834317598026, -6.775152287193681566, -17.89321520033831447 ) ) ;
#11760=CARTESIAN_POINT ( 'NONE',  ( 59.75121349346654398, -13.58877957849836093, -7.404803486908547505 ) ) ;
#11781=CARTESIAN_POINT ( 'NONE',  ( -13.15471766443228141, -4.070564271056700711, -19.15902936687194469 ) ) ;
#11788=VERTEX_POINT ( 'NONE', #32111 ) ;
#11789=DIRECTION ( 'NONE',  ( -0.9908103287288504424, 0.1352586133457951423, 0.000000000000000000 ) ) ;
#11804=ORIENTED_EDGE ( 'NONE', *, *, #25317, .F. ) ;
#11805=CARTESIAN_POINT ( 'NONE',  ( 66.31928500851137187, -14.71576354012722021, -10.39321520033831625 ) ) ;
#11807=CARTESIAN_POINT ( 'NONE',  ( -13.15712544184149202, -4.069566355151700066, -7.629049492614480954 ) ) ;
#11810=CARTESIAN_POINT ( 'NONE',  ( 65.10287265247757205, -0.4742552606671820992, -16.39321520033831447 ) ) ;
#11833=ORIENTED_EDGE ( 'NONE', *, *, #26449, .T. ) ;
#11850=VERTEX_POINT ( 'NONE', #5197 ) ;
#11851=DIRECTION ( 'NONE',  ( 0.1352586133457954198, 0.9908103287288503314, 0.000000000000000000 ) ) ;
#11861=CIRCLE ( 'NONE', #27166, 1.200000000000000178 ) ;
#11896=CARTESIAN_POINT ( 'NONE',  ( 80.91184012100937650, -3.933054092416038650, -19.39321520033831447 ) ) ;
#11900=DIRECTION ( 'NONE',  ( 0.9908103287288504424, -0.1352586133457950590, 0.000000000000000000 ) ) ;
#11931=FACE_OUTER_BOUND ( 'NONE', #37187, .T. ) ;
#11951=LINE ( 'NONE', #32005, #42695 ) ;
#11957=CARTESIAN_POINT ( 'NONE',  ( 61.63318325272354770, -19.46990085680238636, -16.39321520033831447 ) ) ;
#11962=EDGE_CURVE ( 'NONE', #32179, #41326, #22753, .T. ) ;
#11988=CARTESIAN_POINT ( 'NONE',  ( -1.996248100948082360, -6.883391001766379524, -18.88506229808600523 ) ) ;
#11989=CARTESIAN_POINT ( 'NONE',  ( 61.96962176546384882, -13.30635342911269881, -7.742800864598132549 ) ) ;
#12008=CARTESIAN_POINT ( 'NONE',  ( -13.35197469415439464, -5.063788272970252358, -18.19321519141019294 ) ) ;
#12023=CIRCLE ( 'NONE', #21488, 0.5000000000000004441 ) ;
#12034=CARTESIAN_POINT ( 'NONE',  ( 65.52359245923510400, -2.352842260041322575, -8.554674841066066904 ) ) ;
#12064=CARTESIAN_POINT ( 'NONE',  ( -13.55933139336933557, -4.790867379097090151, -17.98576441024524897 ) ) ;
#12066=DIRECTION ( 'NONE',  ( 0.9908103287288504424, -0.1352586133457952255, -0.000000000000000000 ) ) ;
#12076=CIRCLE ( 'NONE', #37546, 6.500000000000000888 ) ;
#12090=CARTESIAN_POINT ( 'NONE',  ( 76.63408154409412987, 1.697290617957241565, -15.89321520033831447 ) ) ;
#12123=DIRECTION ( 'NONE',  ( 0.000000000000000000, 0.000000000000000000, 1.000000000000000000 ) ) ;
#12130=VERTEX_POINT ( 'NONE', #2003 ) ;
#12132=CIRCLE ( 'NONE', #31071, 1.500000000000000888 ) ;
#12155=DIRECTION ( 'NONE',  ( -1.000000000000000000, 0.000000000000000000, 0.000000000000000000 ) ) ;
#12199=DIRECTION ( 'NONE',  ( 0.9908103287288504424, -0.1352586133457952255, -0.000000000000000000 ) ) ;
#12214=DIRECTION ( 'NONE',  ( -0.9908103287288505534, 0.1352586133457944206, 0.000000000000000000 ) ) ;
#12216=CARTESIAN_POINT ( 'NONE',  ( 64.60379348622299744, -13.80859085231287864, -8.919028783932633431 ) ) ;
#12226=EDGE_CURVE ( 'NONE', #259, #6454, #28215, .T. ) ;
#12294=EDGE_CURVE ( 'NONE', #24584, #10084, #14593, .T. ) ;
#12297=LINE ( 'NONE', #19128, #17466 ) ;
#12305=ADVANCED_FACE ( 'NONE', ( #13530 ), #17176, .T. ) ;
#12309=EDGE_CURVE ( 'NONE', #5970, #12356, #30400, .T. ) ;
#12356=VERTEX_POINT ( 'NONE', #6227 ) ;
#12373=CARTESIAN_POINT ( 'NONE',  ( 66.31928500851137187, -14.71576354012722021, -16.39321520033831447 ) ) ;
#12375=AXIS2_PLACEMENT_3D ( 'NONE', #42185, #21649, #10727 ) ;
#12399=CARTESIAN_POINT ( 'NONE',  ( 64.53406607755297841, -2.730567333127841501, -18.66298557222672727 ) ) ;
#12407=AXIS2_PLACEMENT_3D ( 'NONE', #39456, #8219, #4787 ) ;
#12419=EDGE_LOOP ( 'NONE', ( #40291, #15776, #19345, #13720, #7130, #30883 ) ) ;
#12455=DIRECTION ( 'NONE',  ( -0.3127730236694426513, 0.9498278979187093629, 0.000000000000000000 ) ) ;
#12459=CARTESIAN_POINT ( 'NONE',  ( -13.00223655648873589, -4.133127502629707628, -19.24873805723332865 ) ) ;
#12510=LINE ( 'NONE', #19341, #29203 ) ;
#12519=CARTESIAN_POINT ( 'NONE',  ( 59.62174278132244609, -14.86814543204979344, -8.593215200338315540 ) ) ;
#12533=ORIENTED_EDGE ( 'NONE', *, *, #27184, .F. ) ;
#12542=CARTESIAN_POINT ( 'NONE',  ( -13.78505786849281911, -3.796669023460694792, -17.89321520033831447 ) ) ;
#12560=AXIS2_PLACEMENT_3D ( 'NONE', #15726, #6134, #33024 ) ;
#12567=CARTESIAN_POINT ( 'NONE',  ( 75.14134903615895666, -42.50702760616825771, -10.39321520033831625 ) ) ;
#12613=FACE_OUTER_BOUND ( 'NONE', #7976, .T. ) ;
#12630=CARTESIAN_POINT ( 'NONE',  ( 64.64508731025817667, -2.688136943189093575, -18.61997050879359250 ) ) ;
#12634=CARTESIAN_POINT ( 'NONE',  ( -1.910975223132118872, -6.857719673119084369, -7.986702415358247542 ) ) ;
#12668=DIRECTION ( 'NONE',  ( -0.9908103287288503314, 0.1352586133457950868, 0.000000000000000000 ) ) ;
#12672=EDGE_CURVE ( 'NONE', #42783, #6454, #37551, .T. ) ;
#12686=CARTESIAN_POINT ( 'NONE',  ( -13.55938949877377020, -4.790790901322431239, -17.98555846284454418 ) ) ;
#12734=CARTESIAN_POINT ( 'NONE',  ( 41.72636039845269096, -11.37347657059392070, -17.89321520033831447 ) ) ;
#12743=TOROIDAL_SURFACE ( 'NONE', #44054, 33.80000000000000426, 1.199999999999999956 ) ;
#12750=DIRECTION ( 'NONE',  ( 0.000000000000000000, 0.000000000000000000, -1.000000000000000000 ) ) ;
#12784=ADVANCED_FACE ( 'NONE', ( #8060 ), #25618, .F. ) ;
#12798=DIRECTION ( 'NONE',  ( -0.1352586133457944206, -0.9908103287288505534, 0.000000000000000000 ) ) ;
#12806=DIRECTION ( 'NONE',  ( 0.000000000000000000, 0.000000000000000000, 1.000000000000000000 ) ) ;
#12819=EDGE_CURVE ( 'NONE', #27420, #38550, #14453, .T. ) ;
#12854=CARTESIAN_POINT ( 'NONE',  ( 64.04848551113317967, -2.916203086156882840, -18.83592047541311132 ) ) ;
#12858=ORIENTED_EDGE ( 'NONE', *, *, #17794, .T. ) ;
#12889=CARTESIAN_POINT ( 'NONE',  ( 67.19031194842951038, -1.707697914625855296, -14.39321520033831625 ) ) ;
#12898=CARTESIAN_POINT ( 'NONE',  ( 67.96085940327634489, -0.5773760052095162632, -10.39321520033831447 ) ) ;
#12899=PLANE ( 'NONE',  #28957 ) ;
#12903=ORIENTED_EDGE ( 'NONE', *, *, #44280, .F. ) ;
#12920=CARTESIAN_POINT ( 'NONE',  ( 55.68041887817022939, -39.85035523279287162, -9.393215200338314474 ) ) ;
#12923=VERTEX_POINT ( 'NONE', #37148 ) ;
#12949=VECTOR ( 'NONE', #36134, 1000.000000000000000 ) ;
#12967=ORIENTED_EDGE ( 'NONE', *, *, #16682, .F. ) ;
#12986=EDGE_LOOP ( 'NONE', ( #29706, #33431, #10292, #20383 ) ) ;
#13024=EDGE_LOOP ( 'NONE', ( #1427, #36504, #26738, #7863, #75 ) ) ;
#13025=LINE ( 'NONE', #16445, #36167 ) ;
#13047=CARTESIAN_POINT ( 'NONE',  ( -7.917624645353497748, -12.21642755857638818, -19.39321520033831447 ) ) ;
#13104=ORIENTED_EDGE ( 'NONE', *, *, #5695, .T. ) ;
#13107=VECTOR ( 'NONE', #19971, 1000.000000000000000 ) ;
#13115=LINE ( 'NONE', #27474, #42064 ) ;
#13116=AXIS2_PLACEMENT_3D ( 'NONE', #8845, #40541, #9302 ) ;
#13117=CARTESIAN_POINT ( 'NONE',  ( 68.08062758086367694, -0.7900929402678026348, -10.39321520033831625 ) ) ;
#13130=DIRECTION ( 'NONE',  ( 0.000000000000000000, 0.000000000000000000, -1.000000000000000000 ) ) ;
#13151=VERTEX_POINT ( 'NONE', #204 ) ;
#13166=CARTESIAN_POINT ( 'NONE',  ( -13.78505786849281911, -3.796669023460696124, -19.39321520033831447 ) ) ;
#13189=EDGE_CURVE ( 'NONE', #39449, #18952, #39395, .T. ) ;
#13194=FACE_OUTER_BOUND ( 'NONE', #42927, .T. ) ;
#13240=EDGE_CURVE ( 'NONE', #37616, #34939, #19736, .T. ) ;
#13271=CIRCLE ( 'NONE', #27104, 6.000000000000000888 ) ;
#13279=PLANE ( 'NONE',  #16443 ) ;
#13283=DIRECTION ( 'NONE',  ( 0.000000000000000000, 0.000000000000000000, -1.000000000000000000 ) ) ;
#13316=ORIENTED_EDGE ( 'NONE', *, *, #6698, .F. ) ;
#13324=ORIENTED_EDGE ( 'NONE', *, *, #25101, .T. ) ;
#13329=EDGE_CURVE ( 'NONE', #11788, #37616, #42166, .T. ) ;
#13336=CARTESIAN_POINT ( 'NONE',  ( 61.00493324624891756, -4.079101092950570440, -7.393215200338313586 ) ) ;
#13373=ORIENTED_EDGE ( 'NONE', *, *, #41494, .T. ) ;
#13378=CIRCLE ( 'NONE', #32983, 6.000000000000005329 ) ;
#13405=ORIENTED_EDGE ( 'NONE', *, *, #26777, .F. ) ;
#13416=DIRECTION ( 'NONE',  ( 0.9908103287288504424, -0.1352586133457958084, 0.000000000000000000 ) ) ;
#13422=CARTESIAN_POINT ( 'NONE',  ( 9.052690036452151645, -4.182915634381243919, -8.893215200338314474 ) ) ;
#13428=ORIENTED_EDGE ( 'NONE', *, *, #44692, .F. ) ;
#13482=( BOUNDED_SURFACE ( )  B_SPLINE_SURFACE ( 3, 2, ( 
 ( #15405, #32490, #11760 ),
 ( #15631, #43451, #35686 ),
 ( #812, #18599, #29081 ),
 ( #42778, #39349, #11989 ),
 ( #25447, #4230, #8117 ),
 ( #29535, #18149, #29309 ),
 ( #28643, #25670, #39575 ),
 ( #1265, #22018, #14731 ),
 ( #42993, #4461, #1037 ),
 ( #7653, #15175, #12216 ),
 ( #42549, #11310, #25220 ),
 ( #8338, #38884, #43222 ),
 ( #7885, #22238, #39119 ),
 ( #18382, #25890, #4678 ),
 ( #35912, #1483, #22464 ),
 ( #36358, #32270, #36135 ) ),
 .UNSPECIFIED., .F., .F., .T. ) 
 B_SPLINE_SURFACE_WITH_KNOTS ( ( 4, 2, 2, 2, 2, 2, 2, 4 ),
 ( 3, 3 ),
 ( 0.000000000000000000, 0.001721956341060625019, 0.002582934511590937419, 0.003443912682121250037, 0.004304890852651562655, 0.005165869023181874839, 0.006026847193712187023, 0.006887825364242500074 ),
 ( 0.000000000000000000, 1.000000000000000000 ),
 .UNSPECIFIED. ) 
 GEOMETRIC_REPRESENTATION_ITEM ( )  RATIONAL_B_SPLINE_SURFACE ( (
 ( 1.000000000000000000, 0.7145271066604784727, 1.000000000000000000),
 ( 1.000000000000000000, 0.7222084595711586452, 1.000000000000000000),
 ( 1.000000000000000000, 0.7248469248598453651, 1.000000000000000000),
 ( 1.000000000000000000, 0.7198061150658591201, 1.000000000000000000),
 ( 1.000000000000000000, 0.7166464354070819498, 1.000000000000000000),
 ( 1.000000000000000000, 0.7075576805112285816, 1.000000000000000000),
 ( 1.000000000000000000, 0.7016223805004251357, 1.000000000000000000),
 ( 1.000000000000000000, 0.6870357897293317695, 1.000000000000000000),
 ( 1.000000000000000000, 0.6784576229549662552, 1.000000000000000000),
 ( 1.000000000000000000, 0.6592514108187733646, 1.000000000000000000),
 ( 1.000000000000000000, 0.6485859927021864202, 1.000000000000000000),
 ( 1.000000000000000000, 0.6253175026863306840, 1.000000000000000000),
 ( 1.000000000000000000, 0.6127418264104756984, 1.000000000000000000),
 ( 1.000000000000000000, 0.5864433665304108478, 1.000000000000000000),
 ( 1.000000000000000000, 0.5726514202820954802, 1.000000000000000000),
 ( 1.000000000000000000, 0.5583088333832483263, 1.000000000000000000) ) ) 
 REPRESENTATION_ITEM ( '' )  SURFACE ( )  );
#13493=FACE_OUTER_BOUND ( 'NONE', #26819, .T. ) ;
#13497=ORIENTED_EDGE ( 'NONE', *, *, #32531, .T. ) ;
#13500=EDGE_CURVE ( 'NONE', #27420, #1626, #12510, .T. ) ;
#13503=CARTESIAN_POINT ( 'NONE',  ( 59.36680634945872725, -12.84644995903807896, -17.39321520033831447 ) ) ;
#13524=DIRECTION ( 'NONE',  ( 0.1352586133457952255, 0.9908103287288504424, 0.000000000000000000 ) ) ;
#13530=FACE_OUTER_BOUND ( 'NONE', #14808, .T. ) ;
#13532=ORIENTED_EDGE ( 'NONE', *, *, #28069, .F. ) ;
#13551=TOROIDAL_SURFACE ( 'NONE', #31726, 4.500000000000000000, 1.500000000000000000 ) ;
#13566=CARTESIAN_POINT ( 'NONE',  ( 74.82520252044861309, -48.51951888521425360, -10.39321520033831625 ) ) ;
#13583=CARTESIAN_POINT ( 'NONE',  ( 78.93021946355167984, -3.662536865724447921, -19.39321520033831447 ) ) ;
#13627=EDGE_CURVE ( 'NONE', #40326, #511, #34277, .T. ) ;
#13630=DIRECTION ( 'NONE',  ( -0.9908103287288504424, 0.1352586133457950035, 0.000000000000000000 ) ) ;
#13648=CIRCLE ( 'NONE', #44962, 1.499999999999998002 ) ;
#13672=DIRECTION ( 'NONE',  ( 0.9908103287288504424, -0.1352586133457951700, 0.000000000000000000 ) ) ;
#13702=AXIS2_PLACEMENT_3D ( 'NONE', #6325, #41225, #44642 ) ;
#13706=CARTESIAN_POINT ( 'NONE',  ( 41.72636039845269096, -11.37347657059392070, -19.39321520033831447 ) ) ;
#13715=CARTESIAN_POINT ( 'NONE',  ( 61.25533248984433499, -12.48000644236081058, -9.603275126499889680 ) ) ;
#13719=ORIENTED_EDGE ( 'NONE', *, *, #32534, .T. ) ;
#13720=ORIENTED_EDGE ( 'NONE', *, *, #32799, .T. ) ;
#13725=CARTESIAN_POINT ( 'NONE',  ( 59.39246203831174853, -12.83800168394059682, -17.39321520033831447 ) ) ;
#13734=ORIENTED_EDGE ( 'NONE', *, *, #469, .T. ) ;
#13735=ADVANCED_FACE ( 'NONE', ( #25407 ), #39079, .T. ) ;
#13747=CARTESIAN_POINT ( 'NONE',  ( 59.78685257969306122, -14.81377569729345822, -19.38480234211904119 ) ) ;
#13770=FACE_OUTER_BOUND ( 'NONE', #32659, .T. ) ;
#13777=DIRECTION ( 'NONE',  ( -2.312964634635740689E-15, 0.000000000000000000, 1.000000000000000000 ) ) ;
#13795=CARTESIAN_POINT ( 'NONE',  ( 75.14134903615895666, -42.50702760616825771, -15.89321520033831447 ) ) ;
#13800=CARTESIAN_POINT ( 'NONE',  ( 77.44400397045842510, -3.459648945705700473, -10.39321520033831625 ) ) ;
#13831=CARTESIAN_POINT ( 'NONE',  ( 62.35177615844777677, -12.50551974594107740, -16.84622691350345036 ) ) ;
#13836=DIRECTION ( 'NONE',  ( 0.000000000000000000, 0.000000000000000000, -1.000000000000000000 ) ) ;
#13850=VECTOR ( 'NONE', #16659, 999.9999999999998863 ) ;
#13858=EDGE_LOOP ( 'NONE', ( #41512, #20507, #10566, #39269 ) ) ;
#13867=FACE_OUTER_BOUND ( 'NONE', #27920, .T. ) ;
#13880=CARTESIAN_POINT ( 'NONE',  ( -13.90346623771332801, -4.337920405660049994, -8.734217232838743072 ) ) ;
#13887=ADVANCED_FACE ( 'NONE', ( #20309 ), #5925, .T. ) ;
#13914=DIRECTION ( 'NONE',  ( 0.000000000000000000, 0.000000000000000000, 1.000000000000000000 ) ) ;
#13922=( BOUNDED_CURVE ( )  B_SPLINE_CURVE ( 3, ( #25066, #39188, #11161, #21415 ),
 .UNSPECIFIED., .F., .T. ) 
 B_SPLINE_CURVE_WITH_KNOTS ( ( 4, 4 ),
 ( 1.522649623061655300, 1.570796326794896558 ),
 .UNSPECIFIED. ) 
 CURVE ( )  GEOMETRIC_REPRESENTATION_ITEM ( )  RATIONAL_B_SPLINE_CURVE ( ( 1.000000000000000000, 0.9998068339056410680, 0.9998068339056410680, 1.000000000000000000 ) ) 
 REPRESENTATION_ITEM ( '' )  );
#13953=ORIENTED_EDGE ( 'NONE', *, *, #26428, .T. ) ;
#13961=VERTEX_POINT ( 'NONE', #41731 ) ;
#13980=ORIENTED_EDGE ( 'NONE', *, *, #18106, .F. ) ;
#14020=CYLINDRICAL_SURFACE ( 'NONE', #30804, 10.00000000000000000 ) ;
#14034=EDGE_LOOP ( 'NONE', ( #9053, #44887, #29121, #38334 ) ) ;
#14039=ORIENTED_EDGE ( 'NONE', *, *, #26503, .F. ) ;
#14041=AXIS2_PLACEMENT_3D ( 'NONE', #18006, #24629, #38511 ) ;
#14052=DIRECTION ( 'NONE',  ( 0.000000000000000000, 0.000000000000000000, -1.000000000000000000 ) ) ;
#14083=DIRECTION ( 'NONE',  ( 0.1352586133457950590, 0.9908103287288504424, 0.000000000000000000 ) ) ;
#14101=AXIS2_PLACEMENT_3D ( 'NONE', #27659, #6899, #10114 ) ;
#14107=FACE_OUTER_BOUND ( 'NONE', #11093, .T. ) ;
#14127=CARTESIAN_POINT ( 'NONE',  ( 65.38091086278477349, -15.98735439659152036, -17.11731565370446972 ) ) ;
#14143=ORIENTED_EDGE ( 'NONE', *, *, #32555, .F. ) ;
#14144=ADVANCED_FACE ( 'NONE', ( #42624 ), #19106, .T. ) ;
#14153=ORIENTED_EDGE ( 'NONE', *, *, #25608, .F. ) ;
#14170=EDGE_CURVE ( 'NONE', #38280, #13961, #39782, .T. ) ;
#14190=VERTEX_POINT ( 'NONE', #40237 ) ;
#14201=EDGE_CURVE ( 'NONE', #6624, #24134, #4892, .T. ) ;
#14218=PLANE ( 'NONE',  #26747 ) ;
#14239=CARTESIAN_POINT ( 'NONE',  ( 63.44904766416654951, -14.80807631840393945, -16.90507154904199538 ) ) ;
#14241=EDGE_CURVE ( 'NONE', #33232, #1795, #28440, .T. ) ;
#14318=CARTESIAN_POINT ( 'NONE',  ( 60.53937939559665438, -4.256997083809236138, -17.89321520033831447 ) ) ;
#14348=ORIENTED_EDGE ( 'NONE', *, *, #37558, .F. ) ;
#14356=DIRECTION ( 'NONE',  ( -0.9908103287288504424, 0.1352586133457950590, 0.000000000000000000 ) ) ;
#14418=CARTESIAN_POINT ( 'NONE',  ( 3.060777270043529619, -5.064559853354640317, -19.39321520033831447 ) ) ;
#14424=DIRECTION ( 'NONE',  ( -0.9908103287288504424, 0.1352586133457950590, 0.000000000000000000 ) ) ;
#14447=( BOUNDED_CURVE ( )  B_SPLINE_CURVE ( 3, ( #1067, #38909, #7911, #18174 ),
 .UNSPECIFIED., .F., .F. ) 
 B_SPLINE_CURVE_WITH_KNOTS ( ( 4, 4 ),
 ( 0.9676049211852268961, 1.570796326794895004 ),
 .UNSPECIFIED. ) 
 CURVE ( )  GEOMETRIC_REPRESENTATION_ITEM ( )  RATIONAL_B_SPLINE_CURVE ( ( 1.000000000000000000, 0.9699091404214869039, 0.9699091404214869039, 1.000000000000000000 ) ) 
 REPRESENTATION_ITEM ( '' )  );
#14453=LINE ( 'NONE', #35852, #1498 ) ;
#14470=CARTESIAN_POINT ( 'NONE',  ( 75.95778847736514194, -3.256761025687008537, -12.39321520033831447 ) ) ;
#14547=CARTESIAN_POINT ( 'NONE',  ( -13.43406623181752124, -4.955740180368149339, -8.622168566727538064 ) ) ;
#14552=CARTESIAN_POINT ( 'NONE',  ( -1.145390592550948883, -14.88589425535891841, -19.39321520033831447 ) ) ;
#14554=EDGE_CURVE ( 'NONE', #39376, #6119, #22687, .T. ) ;
#14579=ORIENTED_EDGE ( 'NONE', *, *, #36467, .T. ) ;
#14593=CIRCLE ( 'NONE', #30644, 1.199999999999999512 ) ;
#14606=DIRECTION ( 'NONE',  ( 0.9498278979187093629, 0.3127730236694430954, 0.000000000000000000 ) ) ;
#14611=DIRECTION ( 'NONE',  ( 0.1352586133457954198, 0.9908103287288503314, 0.000000000000000000 ) ) ;
#14627=EDGE_LOOP ( 'NONE', ( #19503, #43879, #7818, #42255 ) ) ;
#14633=CARTESIAN_POINT ( 'NONE',  ( 63.98210704970577467, -13.60563849168870121, -18.23844916413033701 ) ) ;
#14637=ORIENTED_EDGE ( 'NONE', *, *, #28259, .F. ) ;
#14652=ORIENTED_EDGE ( 'NONE', *, *, #6085, .F. ) ;
#14659=VECTOR ( 'NONE', #36574, 1000.000000000000000 ) ;
#14670=PRODUCT_DEFINITION_SHAPE ( 'NONE', 'NONE',  #10357 ) ;
#14673=CARTESIAN_POINT ( 'NONE',  ( 27.78057335388972504, -13.48551096636548330, -8.893215200338314474 ) ) ;
#14686=CARTESIAN_POINT ( 'NONE',  ( 61.93251787845459688, -3.724979762910209935, -19.30861058678017272 ) ) ;
#14695=CARTESIAN_POINT ( 'NONE',  ( 64.15128094833310968, -12.93337738546650861, -10.94975984855463835 ) ) ;
#14717=CARTESIAN_POINT ( 'NONE',  ( 62.93082072131119276, -14.63772337390263978, -9.513022489315044794 ) ) ;
#14721=CARTESIAN_POINT ( 'NONE',  ( 75.95778847736514194, -3.256761025687008537, -7.147228641687434880 ) ) ;
#14727=CARTESIAN_POINT ( 'NONE',  ( 35.67453213195965134, -67.60842401891365228, -18.19321520033831519 ) ) ;
#14728=ADVANCED_FACE ( 'NONE', ( #35141 ), #31737, .F. ) ;
#14731=CARTESIAN_POINT ( 'NONE',  ( 63.78489101950506068, -13.55204749033676848, -8.443300631150968627 ) ) ;
#14740=ADVANCED_FACE ( 'NONE', ( #7802 ), #18516, .F. ) ;
#14765=EDGE_CURVE ( 'NONE', #27202, #16955, #26316, .T. ) ;
#14775=CARTESIAN_POINT ( 'NONE',  ( 46.47434218039879283, -17.93412427487546523, -8.593215200338315540 ) ) ;
#14778=DIRECTION ( 'NONE',  ( 0.1352586133457925055, 0.9908103287288507754, 0.000000000000000000 ) ) ;
#14804=CARTESIAN_POINT ( 'NONE',  ( 65.55333354794366585, -16.16208837894097883, -16.95583544328367154 ) ) ;
#14808=EDGE_LOOP ( 'NONE', ( #33730, #23733, #6585, #293 ) ) ;
#14817=DIRECTION ( 'NONE',  ( 0.9908103287288505534, -0.1352586133457945317, 0.000000000000000000 ) ) ;
#14821=CARTESIAN_POINT ( 'NONE',  ( 80.91184012100937650, -3.933054092416038650, -15.89321520033831447 ) ) ;
#14825=CARTESIAN_POINT ( 'NONE',  ( 62.38855081628511101, -1.739798814707631980, -17.65581714534172519 ) ) ;
#14827=EDGE_CURVE ( 'NONE', #30504, #11410, #3046, .T. ) ;
#14849=AXIS2_PLACEMENT_3D ( 'NONE', #33773, #16470, #41983 ) ;
#14851=DIRECTION ( 'NONE',  ( 0.000000000000000000, 0.000000000000000000, -1.000000000000000000 ) ) ;
#14863=CARTESIAN_POINT ( 'NONE',  ( 62.23965954364709319, -13.31694178448660004, -18.96568801859871911 ) ) ;
#14881=CARTESIAN_POINT ( 'NONE',  ( 65.04066262153794753, -15.49774765191802750, -10.45160382476714922 ) ) ;
#14893=DIRECTION ( 'NONE',  ( 0.1352586133457954198, 0.9908103287288503314, 0.000000000000000000 ) ) ;
#14914=CARTESIAN_POINT ( 'NONE',  ( 62.09114116458580668, -3.664294667776160974, -19.28739984847905831 ) ) ;
#14927=DIRECTION ( 'NONE',  ( -0.9908103287288502203, 0.1352586133457974182, 0.000000000000000000 ) ) ;
#14935=ORIENTED_EDGE ( 'NONE', *, *, #4943, .T. ) ;
#14942=CARTESIAN_POINT ( 'NONE',  ( 63.92618626572875229, -15.01321783771896534, -10.28494218876606858 ) ) ;
#14954=CARTESIAN_POINT ( 'NONE',  ( 60.99435512697144190, -13.32931833351154793, -7.514629966800860927 ) ) ;
#14998=CARTESIAN_POINT ( 'NONE',  ( 63.54424027483572246, -3.108909839411367226, -7.798187301296191976 ) ) ;
#15001=CARTESIAN_POINT ( 'NONE',  ( 66.59991520736690518, -0.05656289534533872482, -16.39321520033831092 ) ) ;
#15024=AXIS2_PLACEMENT_3D ( 'NONE', #27214, #41132, #24454 ) ;
#15029=CARTESIAN_POINT ( 'NONE',  ( 62.28500519901574251, -13.31919971779094070, -18.95210956505300715 ) ) ;
#15038=SURFACE_SIDE_STYLE ('',( #32354 ) ) ;
#15041=CARTESIAN_POINT ( 'NONE',  ( 65.10287265247758626, -0.4742552606671335269, -10.39321520033831625 ) ) ;
#15044=AXIS2_PLACEMENT_3D ( 'NONE', #35543, #4315, #898 ) ;
#15047=CARTESIAN_POINT ( 'NONE',  ( 67.93051324133456603, 0.8441227859799155242, -16.93281709690001335 ) ) ;
#15061=DIRECTION ( 'NONE',  ( -0.9908103287288503314, 0.1352586133457956419, 0.000000000000000000 ) ) ;
#15077=EDGE_LOOP ( 'NONE', ( #14579, #5946, #35987, #24705 ) ) ;
#15084=CARTESIAN_POINT ( 'NONE',  ( 66.12481753886987690, -14.57890275351189402, -16.60867411372743518 ) ) ;
#15095=PRODUCT_DEFINITION_CONTEXT ( 'detailed design', #18372, 'design' ) ;
#15109=ORIENTED_EDGE ( 'NONE', *, *, #3676, .T. ) ;
#15124=LINE ( 'NONE', #18769, #15283 ) ;
#15125=ORIENTED_EDGE ( 'NONE', *, *, #36224, .F. ) ;
#15132=ORIENTED_EDGE ( 'NONE', *, *, #32799, .F. ) ;
#15156=EDGE_CURVE ( 'NONE', #37616, #36955, #13271, .T. ) ;
#15158=EDGE_LOOP ( 'NONE', ( #17802, #41972, #13980, #41905 ) ) ;
#15170=CARTESIAN_POINT ( 'NONE',  ( -13.60420442504482175, -3.877746523608537554, -8.129294934689871965 ) ) ;
#15175=CARTESIAN_POINT ( 'NONE',  ( 64.18188758151919160, -15.10253999624987742, -8.768039431438440445 ) ) ;
#15196=( BOUNDED_SURFACE ( )  B_SPLINE_SURFACE ( 3, 2, ( 
 ( #30025, #24534, #27963 ),
 ( #3548, #41433, #3110 ),
 ( #10630, #20675, #2883 ),
 ( #41207, #41653, #34979 ),
 ( #37765, #40984, #16812 ),
 ( #17463, #21100, #34552 ) ),
 .UNSPECIFIED., .F., .F., .F. ) 
 B_SPLINE_SURFACE_WITH_KNOTS ( ( 4, 2, 4 ),
 ( 3, 3 ),
 ( 3.899122207871039691, 4.305755594127865571, 4.712388980384689674 ),
 ( 0.000000000000000000, 1.000000000000000000 ),
 .UNSPECIFIED. ) 
 GEOMETRIC_REPRESENTATION_ITEM ( )  RATIONAL_B_SPLINE_SURFACE ( (
 ( 1.000000000000000000, 0.5507912154400889104, 1.000000000000000000),
 ( 1.000000000000000000, 0.5736970358664340575, 1.000000000000000000),
 ( 1.000000000000000000, 0.5999889691994200192, 1.000000000000000000),
 ( 1.000000000000000000, 0.6537365690953489406, 1.000000000000000000),
 ( 1.000000000000000000, 0.6811922875906900599, 1.000000000000000000),
 ( 1.000000000000000000, 0.7071067811865480168, 1.000000000000000000) ) ) 
 REPRESENTATION_ITEM ( '' )  SURFACE ( )  );
#15197=CARTESIAN_POINT ( 'NONE',  ( -13.42620672024982476, -3.955390967436159588, -18.90065854372406662 ) ) ;
#15205=DIRECTION ( 'NONE',  ( -0.9908103287288497762, 0.1352586133458010265, 0.000000000000000000 ) ) ;
#15218=ORIENTED_EDGE ( 'NONE', *, *, #33363, .F. ) ;
#15221=CARTESIAN_POINT ( 'NONE',  ( 64.91709923316010133, -47.16693275175630617, -12.39321520033831447 ) ) ;
#15227=DIRECTION ( 'NONE',  ( 0.1352586133457954198, 0.9908103287288503314, 0.000000000000000000 ) ) ;
#15280=AXIS2_PLACEMENT_3D ( 'NONE', #13583, #27493, #20652 ) ;
#15281=CARTESIAN_POINT ( 'NONE',  ( 81.52050388106540879, 0.5255923868638483487, -10.89321520033831447 ) ) ;
#15283=VECTOR ( 'NONE', #32658, 1000.000000000000000 ) ;
#15303=CARTESIAN_POINT ( 'NONE',  ( 64.51132457273423881, -13.77492255257581455, -17.92675206381565189 ) ) ;
#15305=EDGE_CURVE ( 'NONE', #10182, #511, #1126, .T. ) ;
#15334=DIRECTION ( 'NONE',  ( -0.9908103287288504424, 0.1352586133457950868, 0.000000000000000000 ) ) ;
#15364=CARTESIAN_POINT ( 'NONE',  ( 62.30685165342923426, -3.581745535644693224, -19.25472737399296719 ) ) ;
#15373=DIRECTION ( 'NONE',  ( -0.1352586133457950590, -0.9908103287288504424, 0.000000000000000000 ) ) ;
#15405=CARTESIAN_POINT ( 'NONE',  ( 60.06931813437628875, -14.72076136720885309, -8.603412892520120536 ) ) ;
#15408=ORIENTED_EDGE ( 'NONE', *, *, #18053, .F. ) ;
#15410=CARTESIAN_POINT ( 'NONE',  ( 66.16856755279033564, -15.11643429149317619, -10.39321520033831270 ) ) ;
#15429=CARTESIAN_POINT ( 'NONE',  ( 46.47434218039879283, -17.93412427487546523, -19.39321520033831447 ) ) ;
#15449=CARTESIAN_POINT ( 'NONE',  ( -12.68961124276041019, -4.256188596408917668, -7.420957702222477970 ) ) ;
#15470=DIRECTION ( 'NONE',  ( -0.9498278979187094739, -0.3127730236694427068, -0.000000000000000000 ) ) ;
#15479=FACE_OUTER_BOUND ( 'NONE', #9041, .T. ) ;
#15487=CARTESIAN_POINT ( 'NONE',  ( 75.95778847736514194, -3.256761025687008537, -12.39321520033831447 ) ) ;
#15531=CARTESIAN_POINT ( 'NONE',  ( 71.31713442278437753, 2.423123680056944007, -19.39321520033831447 ) ) ;
#15589=ORIENTED_EDGE ( 'NONE', *, *, #3676, .F. ) ;
#15605=VERTEX_POINT ( 'NONE', #37200 ) ;
#15620=CARTESIAN_POINT ( 'NONE',  ( 64.75357039381266588, -13.20363101263777850, -15.30938453869310578 ) ) ;
#15623=CARTESIAN_POINT ( 'NONE',  ( 66.58723489636778936, -20.14619392353143112, -15.89321520033831447 ) ) ;
#15629=CARTESIAN_POINT ( 'NONE',  ( 71.04661719609278236, 0.4415030225992447321, -14.39321520033831625 ) ) ;
#15630=CARTESIAN_POINT ( 'NONE',  ( -2.172448456896171720, -6.936427131018752412, -19.06457999368345924 ) ) ;
#15631=CARTESIAN_POINT ( 'NONE',  ( 60.51500512425220535, -14.57399912981923684, -8.628611073238383611 ) ) ;
#15636=DIRECTION ( 'NONE',  ( 0.000000000000000000, 0.000000000000000000, -1.000000000000000000 ) ) ;
#15658=DIRECTION ( 'NONE',  ( 0.000000000000000000, 0.000000000000000000, -1.000000000000000000 ) ) ;
#15674=CARTESIAN_POINT ( 'NONE',  ( 62.63422871652684876, -3.456519832263517333, -7.588643140964075329 ) ) ;
#15680=ADVANCED_FACE ( 'NONE', ( #2787 ), #40194, .T. ) ;
#15697=DIRECTION ( 'NONE',  ( 0.000000000000000000, 0.000000000000000000, 1.000000000000000000 ) ) ;
#15698=DIRECTION ( 'NONE',  ( 0.3127730236694426513, -0.9498278979187093629, 0.000000000000000000 ) ) ;
#15699=ADVANCED_FACE ( 'NONE', ( #15799 ), #16714, .T. ) ;
#15726=CARTESIAN_POINT ( 'NONE',  ( 35.90261398037149121, 14.17005867477686820, -8.593215200338315540 ) ) ;
#15737=VECTOR ( 'NONE', #29715, 1000.000000000000000 ) ;
#15773=AXIS2_PLACEMENT_3D ( 'NONE', #24469, #31301, #17193 ) ;
#15776=ORIENTED_EDGE ( 'NONE', *, *, #41219, .T. ) ;
#15782=ORIENTED_EDGE ( 'NONE', *, *, #29573, .F. ) ;
#15786=CARTESIAN_POINT ( 'NONE',  ( 66.30459164891361468, -14.82339685155236886, -16.39321520033831447 ) ) ;
#15799=FACE_OUTER_BOUND ( 'NONE', #7082, .T. ) ;
#15801=DIRECTION ( 'NONE',  ( 0.9908103287288504424, -0.1352586133457951423, 0.000000000000000000 ) ) ;
#15811=CARTESIAN_POINT ( 'NONE',  ( 63.00984045858719185, -3.312991842083455207, -19.12743919334240417 ) ) ;
#15816=CARTESIAN_POINT ( 'NONE',  ( 31.16856251326851179, -20.50830283073288030, -18.19321520033831519 ) ) ;
#15822=FACE_OUTER_BOUND ( 'NONE', #1353, .T. ) ;
#15842=EDGE_CURVE ( 'NONE', #11410, #19947, #6448, .T. ) ;
#15858=CARTESIAN_POINT ( 'NONE',  ( 65.99667006149269355, -0.1541283259764877900, -10.39321520033831270 ) ) ;
#15876=CARTESIAN_POINT ( 'NONE',  ( -13.56828337869085210, -4.779084862085888119, -17.89321520033830026 ) ) ;
#15891=CARTESIAN_POINT ( 'NONE',  ( -3.075987277002700804, -7.207016596002322473, -19.39321520033831447 ) ) ;
#15907=CARTESIAN_POINT ( 'NONE',  ( 67.62945316293361486, -0.2852776976338805004, -16.39321520033831447 ) ) ;
#15938=ORIENTED_EDGE ( 'NONE', *, *, #14765, .T. ) ;
#15942=DIRECTION ( 'NONE',  ( -0.9908103287288504424, 0.1352586133457951423, 0.000000000000000000 ) ) ;
#15954=VERTEX_POINT ( 'NONE', #17817 ) ;
#15982=LINE ( 'NONE', #42899, #22668 ) ;
#15997=EDGE_LOOP ( 'NONE', ( #7504, #12533 ) ) ;
#16037=CARTESIAN_POINT ( 'NONE',  ( 64.65425730835187323, -2.684632774272076805, -18.61636701123672921 ) ) ;
#16044=APPLICATION_CONTEXT ( 'automotive_design' ) ;
#16058=ORIENTED_EDGE ( 'NONE', *, *, #5527, .F. ) ;
#16069=CARTESIAN_POINT ( 'NONE',  ( 63.12337091419462354, -3.603895683774054781, -17.39321520033831447 ) ) ;
#16078=CARTESIAN_POINT ( 'NONE',  ( 67.37843845263206788, -0.1674546162330892152, -10.39321520033831625 ) ) ;
#16109=CIRCLE ( 'NONE', #44526, 1.199999999999999512 ) ;
#16124=EDGE_CURVE ( 'NONE', #18680, #29964, #10371, .T. ) ;
#16139=VERTEX_POINT ( 'NONE', #932 ) ;
#16154=ORIENTED_EDGE ( 'NONE', *, *, #40694, .T. ) ;
#16180=DIRECTION ( 'NONE',  ( 0.000000000000000000, 0.000000000000000000, -1.000000000000000000 ) ) ;
#16184=CARTESIAN_POINT ( 'NONE',  ( 60.06931813437629586, -14.72076136720887085, -8.603412892520118760 ) ) ;
#16199=ADVANCED_FACE ( 'NONE', ( #31383 ), #6557, .T. ) ;
#16218=ORIENTED_EDGE ( 'NONE', *, *, #9439, .T. ) ;
#16231=TOROIDAL_SURFACE ( 'NONE', #32216, 8.800000000000000711, 1.199999999999999956 ) ;
#16290=VERTEX_POINT ( 'NONE', #154 ) ;
#16298=CARTESIAN_POINT ( 'NONE',  ( 65.52504830115719869, -2.484121567297625788, -10.46358271731430989 ) ) ;
#16299=ORIENTED_EDGE ( 'NONE', *, *, #20436, .F. ) ;
#16312=CARTESIAN_POINT ( 'NONE',  ( 64.46696884417693241, -15.35047623415474405, -15.89321305673442986 ) ) ;
#16401=VERTEX_POINT ( 'NONE', #17711 ) ;
#16443=AXIS2_PLACEMENT_3D ( 'NONE', #6660, #44747, #21006 ) ;
#16445=CARTESIAN_POINT ( 'NONE',  ( 71.62928943233082180, 0.3619606153155430217, -19.39321520033831447 ) ) ;
#16463=VERTEX_POINT ( 'NONE', #21580 ) ;
#16466=AXIS2_PLACEMENT_3D ( 'NONE', #31335, #2852, #38181 ) ;
#16470=DIRECTION ( 'NONE',  ( 0.000000000000000000, 0.000000000000000000, -1.000000000000000000 ) ) ;
#16488=TOROIDAL_SURFACE ( 'NONE', #24484, 6.500000000000000000, 1.500000000000000000 ) ;
#16493=CARTESIAN_POINT ( 'NONE',  ( 31.33087284928346605, -19.31933043625826585, -19.39321520033831447 ) ) ;
#16547=DIRECTION ( 'NONE',  ( 0.000000000000000000, 0.000000000000000000, 1.000000000000000000 ) ) ;
#16593=CARTESIAN_POINT ( 'NONE',  ( 63.74703025577719018, -40.95155355269160680, -10.89321520033831447 ) ) ;
#16659=DIRECTION ( 'NONE',  ( 0.6049664196031393493, -0.7962509850245451659, 0.000000000000000000 ) ) ;
#16682=EDGE_CURVE ( 'NONE', #9245, #39715, #11861, .T. ) ;
#16709=EDGE_CURVE ( 'NONE', #3183, #33968, #35853, .T. ) ;
#16714=CYLINDRICAL_SURFACE ( 'NONE', #25659, 1.500000000000001332 ) ;
#16720=EDGE_LOOP ( 'NONE', ( #34362, #35711, #6677, #14637 ) ) ;
#16733=AXIS2_PLACEMENT_3D ( 'NONE', #34236, #13283, #3010 ) ;
#16742=ADVANCED_FACE ( 'NONE', ( #40716 ), #16231, .T. ) ;
#16756=CARTESIAN_POINT ( 'NONE',  ( 62.70662433455723317, -3.428858449946674103, -7.602483789130480396 ) ) ;
#16810=ORIENTED_EDGE ( 'NONE', *, *, #17527, .F. ) ;
#16812=CARTESIAN_POINT ( 'NONE',  ( 61.98298312043991132, -3.705371713990854854, -7.393215200338315363 ) ) ;
#16814=CARTESIAN_POINT ( 'NONE',  ( 31.16856251326852956, -20.50830283073288385, -8.593215200338315540 ) ) ;
#16823=FACE_OUTER_BOUND ( 'NONE', #44337, .T. ) ;
#16826=ORIENTED_EDGE ( 'NONE', *, *, #19491, .T. ) ;
#16848=CARTESIAN_POINT ( 'NONE',  ( 27.78057335388972504, -13.48551096636548330, -8.893215200338314474 ) ) ;
#16850=ORIENTED_EDGE ( 'NONE', *, *, #29281, .T. ) ;
#16867=ORIENTED_EDGE ( 'NONE', *, *, #23670, .F. ) ;
#16916=CARTESIAN_POINT ( 'NONE',  ( 61.28923319885182508, -12.47826754884034983, -9.611157264325234095 ) ) ;
#16928=CARTESIAN_POINT ( 'NONE',  ( 71.31713442278437753, 2.423123680056944007, -15.89321520033831447 ) ) ;
#16955=VERTEX_POINT ( 'NONE', #13800 ) ;
#16981=ORIENTED_EDGE ( 'NONE', *, *, #13329, .T. ) ;
#16982=EDGE_CURVE ( 'NONE', #42225, #17020, #21753, .T. ) ;
#16996=DIRECTION ( 'NONE',  ( -0.1352586133457952255, -0.9908103287288504424, 0.000000000000000000 ) ) ;
#17002=ORIENTED_EDGE ( 'NONE', *, *, #490, .F. ) ;
#17010=DIRECTION ( 'NONE',  ( -0.3127730236694482580, 0.9498278979187074755, 0.000000000000000000 ) ) ;
#17020=VERTEX_POINT ( 'NONE', #28602 ) ;
#17024=VECTOR ( 'NONE', #23912, 1000.000000000000114 ) ;
#17043=ADVANCED_FACE ( 'NONE', ( #31781 ), #14020, .T. ) ;
#17069=CARTESIAN_POINT ( 'NONE',  ( 61.63318325272354770, -19.46990085680238636, -14.39321520033831625 ) ) ;
#17078=CARTESIAN_POINT ( 'NONE',  ( 71.04661719609278236, 0.4415030225992447321, -19.39321520033831447 ) ) ;
#17084=DIRECTION ( 'NONE',  ( -0.4225728684367167642, 0.9063289528979890930, 0.000000000000000000 ) ) ;
#17104=( GEOMETRIC_REPRESENTATION_CONTEXT ( 3 ) GLOBAL_UNCERTAINTY_ASSIGNED_CONTEXT ( ( #7345 ) ) GLOBAL_UNIT_ASSIGNED_CONTEXT ( ( #8867, #11616, #18464 ) ) REPRESENTATION_CONTEXT ( 'NONE', 'WORKASPACE' ) );
#17106=AXIS2_PLACEMENT_3D ( 'NONE', #3830, #34393, #20287 ) ;
#17126=EDGE_CURVE ( 'NONE', #39715, #35887, #7968, .T. ) ;
#17140=DIRECTION ( 'NONE',  ( 0.9063289528979890930, 0.4225728684367167087, 0.000000000000000000 ) ) ;
#17145=ORIENTED_EDGE ( 'NONE', *, *, #31701, .T. ) ;
#17149=CARTESIAN_POINT ( 'NONE',  ( 74.82520252044861309, -48.51951888521425360, -14.39321520033831625 ) ) ;
#17168=VERTEX_POINT ( 'NONE', #1885 ) ;
#17176=CYLINDRICAL_SURFACE ( 'NONE', #36450, 1.199999999999999067 ) ;
#17178=ORIENTED_EDGE ( 'NONE', *, *, #43477, .F. ) ;
#17193=DIRECTION ( 'NONE',  ( 0.9908103287288505534, -0.1352586133457945317, 0.000000000000000000 ) ) ;
#17201=FACE_OUTER_BOUND ( 'NONE', #39289, .T. ) ;
#17202=CARTESIAN_POINT ( 'NONE',  ( 62.39342502807065216, -3.548534728824127793, -7.543532614991891982 ) ) ;
#17238=ORIENTED_EDGE ( 'NONE', *, *, #10709, .F. ) ;
#17245=ADVANCED_FACE ( 'NONE', ( #23108 ), #36544, .F. ) ;
#17259=CARTESIAN_POINT ( 'NONE',  ( 70.97035005826802490, 2.261436620216122240, -10.39321520033832158 ) ) ;
#17267=DIRECTION ( 'NONE',  ( 1.000000000000000000, 0.000000000000000000, 0.000000000000000000 ) ) ;
#17289=DIRECTION ( 'NONE',  ( -1.000000000000000000, 0.000000000000000000, 0.000000000000000000 ) ) ;
#17316=CYLINDRICAL_SURFACE ( 'NONE', #19304, 6.000000000000000888 ) ;
#17352=CARTESIAN_POINT ( 'NONE',  ( -7.923679509334008664, -5.078949698970065540, -17.89321520033831447 ) ) ;
#17359=CARTESIAN_POINT ( 'NONE',  ( 62.94933249576302359, -12.59472958831572775, -10.20703604984677959 ) ) ;
#17370=CARTESIAN_POINT ( 'NONE',  ( 31.33087284928346605, -19.31933043625826230, -7.393215200338315363 ) ) ;
#17372=DIRECTION ( 'NONE',  ( -0.9908103287288505534, 0.1352586133457950590, 0.000000000000000000 ) ) ;
#17418=DIRECTION ( 'NONE',  ( 0.000000000000000000, 0.000000000000000000, -1.000000000000000000 ) ) ;
#17463=CARTESIAN_POINT ( 'NONE',  ( 59.90552009294157898, -2.897503654462289191, -8.893215200338314474 ) ) ;
#17466=VECTOR ( 'NONE', #29613, 1000.000000000000000 ) ;
#17471=CARTESIAN_POINT ( 'NONE',  ( 63.41276417961783096, -12.69524715595927589, -16.33464570172938224 ) ) ;
#17512=ORIENTED_EDGE ( 'NONE', *, *, #42420, .F. ) ;
#17527=EDGE_CURVE ( 'NONE', #9245, #24192, #13922, .T. ) ;
#17537=EDGE_CURVE ( 'NONE', #37929, #11150, #10173, .T. ) ;
#17551=CARTESIAN_POINT ( 'NONE',  ( 60.06931813437628875, -14.72076136720885309, -18.18301750815651374 ) ) ;
#17567=VERTEX_POINT ( 'NONE', #35528 ) ;
#17580=ORIENTED_EDGE ( 'NONE', *, *, #8493, .F. ) ;
#17631=AXIS2_PLACEMENT_3D ( 'NONE', #21863, #35758, #33548 ) ;
#17638=CYLINDRICAL_SURFACE ( 'NONE', #21549, 1.499999999999998002 ) ;
#17711=CARTESIAN_POINT ( 'NONE',  ( -7.917624645353497748, -12.21642755857638818, -18.19321520033831519 ) ) ;
#17740=EDGE_CURVE ( 'NONE', #9071, #43660, #35018, .T. ) ;
#17772=CARTESIAN_POINT ( 'NONE',  ( 60.37455426411234782, -13.41643124914782703, -19.35299115515521606 ) ) ;
#17786=DIRECTION ( 'NONE',  ( -0.9908103287288504424, 0.1352586133457950590, 0.000000000000000000 ) ) ;
#17794=EDGE_CURVE ( 'NONE', #30249, #35231, #42492, .T. ) ;
#17797=EDGE_CURVE ( 'NONE', #41268, #16139, #44683, .T. ) ;
#17802=ORIENTED_EDGE ( 'NONE', *, *, #38102, .F. ) ;
#17816=ORIENTED_EDGE ( 'NONE', *, *, #10663, .F. ) ;
#17817=CARTESIAN_POINT ( 'NONE',  ( 74.43213512091445239, -36.61236768192972590, -14.39321520033831625 ) ) ;
#17847=CARTESIAN_POINT ( 'NONE',  ( 75.63675420052337017, -42.57465691284114939, -10.89321520033831447 ) ) ;
#17891=CIRCLE ( 'NONE', #44136, 12.50000000000000178 ) ;
#17918=CARTESIAN_POINT ( 'NONE',  ( 62.66980483302768334, -12.54647196691845323, -16.71198379459248429 ) ) ;
#17922=CARTESIAN_POINT ( 'NONE',  ( 81.52050388106540879, 0.5255923868638483487, -15.89321520033831447 ) ) ;
#17934=AXIS2_PLACEMENT_3D ( 'NONE', #24630, #10731, #42635 ) ;
#17961=ORIENTED_EDGE ( 'NONE', *, *, #41910, .T. ) ;
#17969=CARTESIAN_POINT ( 'NONE',  ( 65.41257106814472877, -15.47412461924279725, -16.39321520033831447 ) ) ;
#17991=ORIENTED_EDGE ( 'NONE', *, *, #35379, .T. ) ;
#18006=CARTESIAN_POINT ( 'NONE',  ( 2.181596283295915484, -11.50482699009217669, -8.893215200338314474 ) ) ;
#18008=DIRECTION ( 'NONE',  ( 0.000000000000000000, 0.000000000000000000, -1.000000000000000000 ) ) ;
#18053=EDGE_CURVE ( 'NONE', #2987, #39376, #13378, .T. ) ;
#18085=VERTEX_POINT ( 'NONE', #27476 ) ;
#18086=FACE_OUTER_BOUND ( 'NONE', #35555, .T. ) ;
#18106=EDGE_CURVE ( 'NONE', #1972, #27420, #19184, .T. ) ;
#18111=VERTEX_POINT ( 'NONE', #32825 ) ;
#18115=CARTESIAN_POINT ( 'NONE',  ( 64.40208719633689327, -13.04080931321579406, -11.16048930627172808 ) ) ;
#18143=EDGE_CURVE ( 'NONE', #1626, #43799, #4592, .T. ) ;
#18149=CARTESIAN_POINT ( 'NONE',  ( 62.73792221385235734, -14.56781324038501602, -8.049265019886933104 ) ) ;
#18174=CARTESIAN_POINT ( 'NONE',  ( 59.90552009294157898, -2.897503654462289191, -17.89321520033831447 ) ) ;
#18192=CARTESIAN_POINT ( 'NONE',  ( -12.36826994950263980, -4.374949827406455327, -7.393215200338315363 ) ) ;
#18211=DIRECTION ( 'NONE',  ( 0.000000000000000000, 0.000000000000000000, -1.000000000000000000 ) ) ;
#18217=ORIENTED_EDGE ( 'NONE', *, *, #15156, .T. ) ;
#18219=CARTESIAN_POINT ( 'NONE',  ( 64.46696884418977902, -15.35047623416358142, -10.89321734395795893 ) ) ;
#18223=CARTESIAN_POINT ( 'NONE',  ( 66.01377532187956376, -14.50698776528348688, -16.72205822936306063 ) ) ;
#18246=DIRECTION ( 'NONE',  ( -1.000000000000000000, 0.000000000000000000, 0.000000000000000000 ) ) ;
#18253=CYLINDRICAL_SURFACE ( 'NONE', #22941, 1.199999999999999512 ) ;
#18257=DIRECTION ( 'NONE',  ( -0.9908103287288504424, 0.1352586133457950035, 0.000000000000000000 ) ) ;
#18273=ORIENTED_EDGE ( 'NONE', *, *, #8860, .F. ) ;
#18297=DIRECTION ( 'NONE',  ( 0.000000000000000000, 0.000000000000000000, 1.000000000000000000 ) ) ;
#18311=LINE ( 'NONE', #21952, #9182 ) ;
#18320=LINE ( 'NONE', #42941, #24036 ) ;
#18333=CARTESIAN_POINT ( 'NONE',  ( 60.53937939559665438, -4.256997083809236138, -19.39321520033831447 ) ) ;
#18340=VECTOR ( 'NONE', #11851, 1000.000000000000114 ) ;
#18342=CARTESIAN_POINT ( 'NONE',  ( 65.16811225466804558, -13.42767900044409579, -11.91060832829492711 ) ) ;
#18355=DIRECTION ( 'NONE',  ( 0.000000000000000000, 0.000000000000000000, -1.000000000000000000 ) ) ;
#18365=EDGE_CURVE ( 'NONE', #17168, #9021, #11271, .T. ) ;
#18372=APPLICATION_CONTEXT ( 'automotive_design' ) ;
#18373=LINE ( 'NONE', #25439, #1833 ) ;
#18380=AXIS2_PLACEMENT_3D ( 'NONE', #30084, #9107, #2707 ) ;
#18382=CARTESIAN_POINT ( 'NONE',  ( 64.51296881898170454, -15.37845651475741349, -10.94392415253807727 ) ) ;
#18409=AXIS2_PLACEMENT_3D ( 'NONE', #20098, #226, #33983 ) ;
#18422=EDGE_CURVE ( 'NONE', #35546, #7942, #38086, .T. ) ;
#18427=CARTESIAN_POINT ( 'NONE',  ( 65.35735161495482259, -2.416243571375609189, -8.473654787043400916 ) ) ;
#18431=EDGE_CURVE ( 'NONE', #38238, #854, #23736, .T. ) ;
#18435=AXIS2_PLACEMENT_3D ( 'NONE', #15531, #12798, #26699 ) ;
#18450=LINE ( 'NONE', #42617, #35537 ) ;
#18464=( NAMED_UNIT ( * ) SI_UNIT ( $, .STERADIAN. ) SOLID_ANGLE_UNIT ( ) );
#18466=CARTESIAN_POINT ( 'NONE',  ( 69.69189222815028018, -41.76310523276638520, -15.89321520033831447 ) ) ;
#18474=CARTESIAN_POINT ( 'NONE',  ( 66.56178116512437271, 0.2059559948650140082, -15.23405342170197940 ) ) ;
#18475=ORIENTED_EDGE ( 'NONE', *, *, #9456, .T. ) ;
#18516=PLANE ( 'NONE',  #42363 ) ;
#18527=CIRCLE ( 'NONE', #326, 1.199999999999999067 ) ;
#18533=ADVANCED_FACE ( 'NONE', ( #19911 ), #40206, .T. ) ;
#18536=DIRECTION ( 'NONE',  ( 0.000000000000000000, 0.000000000000000000, 1.000000000000000000 ) ) ;
#18575=DIRECTION ( 'NONE',  ( 0.1352586133457950590, 0.9908103287288504424, 0.000000000000000000 ) ) ;
#18585=CARTESIAN_POINT ( 'NONE',  ( 61.55121550910386219, -14.46605081255136049, -8.868903071359692802 ) ) ;
#18593=CARTESIAN_POINT ( 'NONE',  ( 65.00050459711196993, -13.33302880096658249, -15.05917699090357509 ) ) ;
#18599=CARTESIAN_POINT ( 'NONE',  ( 61.15360158040112282, -14.46165722119120822, -7.573710289374333549 ) ) ;
#18605=FACE_OUTER_BOUND ( 'NONE', #4707, .T. ) ;
#18627=ADVANCED_FACE ( 'NONE', ( #20147 ), #27878, .F. ) ;
#18643=EDGE_CURVE ( 'NONE', #42460, #39949, #5988, .T. ) ;
#18646=DIRECTION ( 'NONE',  ( 0.9498278979187094739, 0.3127730236694427068, -0.000000000000000000 ) ) ;
#18664=ORIENTED_EDGE ( 'NONE', *, *, #19476, .T. ) ;
#18680=VERTEX_POINT ( 'NONE', #27208 ) ;
#18682=CARTESIAN_POINT ( 'NONE',  ( 65.10287265247757205, -0.4742552606671820992, -16.39321520033831447 ) ) ;
#18699=ORIENTED_EDGE ( 'NONE', *, *, #25117, .F. ) ;
#18707=AXIS2_PLACEMENT_3D ( 'NONE', #36599, #5375, #19292 ) ;
#18730=CARTESIAN_POINT ( 'NONE',  ( -13.78505786849295411, -3.796669023460440329, -18.09332867002095213 ) ) ;
#18738=CIRCLE ( 'NONE', #36194, 1.199999999999999512 ) ;
#18740=DIRECTION ( 'NONE',  ( -0.3127730236694430399, 0.9498278979187092519, 0.000000000000000000 ) ) ;
#18769=CARTESIAN_POINT ( 'NONE',  ( 59.44377208703740223, -12.82110557137145967, -19.39321520033831447 ) ) ;
#18783=DIRECTION ( 'NONE',  ( 0.000000000000000000, 0.000000000000000000, -1.000000000000000000 ) ) ;
#18794=CARTESIAN_POINT ( 'NONE',  ( 54.86886719809545809, -45.79521720516596872, -17.39321520033831447 ) ) ;
#18814=DIRECTION ( 'NONE',  ( -0.1352586133457952255, -0.9908103287288504424, 0.000000000000000000 ) ) ;
#18818=CARTESIAN_POINT ( 'NONE',  ( -1.769543856513131397, -6.815240831730628557, -18.52879468264121243 ) ) ;
#18819=CARTESIAN_POINT ( 'NONE',  ( 60.37068618338318515, -13.41750073646542241, -7.433261549074098973 ) ) ;
#18845=EDGE_LOOP ( 'NONE', ( #30530, #3, #25991, #13324 ) ) ;
#18862=CARTESIAN_POINT ( 'NONE',  ( -13.32377113153209436, -5.100909530930224811, -7.393215200338312698 ) ) ;
#18863=CARTESIAN_POINT ( 'NONE',  ( 2.384484203314607420, -10.01861149699890063, -19.39321520033831447 ) ) ;
#18865=CARTESIAN_POINT ( 'NONE',  ( 67.71887983560293378, -0.3398796721086269068, -16.39321520033832158 ) ) ;
#18885=CIRCLE ( 'NONE', #39266, 1.499999999999998002 ) ;
#18903=EDGE_CURVE ( 'NONE', #9021, #36955, #37266, .T. ) ;
#18920=EDGE_CURVE ( 'NONE', #11018, #9245, #31861, .T. ) ;
#18930=AXIS2_PLACEMENT_3D ( 'NONE', #5301, #4623, #12155 ) ;
#18943=ORIENTED_EDGE ( 'NONE', *, *, #20045, .T. ) ;
#18952=VERTEX_POINT ( 'NONE', #497 ) ;
#18987=CARTESIAN_POINT ( 'NONE',  ( 35.90261398037149121, 14.17005867477686820, -19.39321520033831447 ) ) ;
#18995=ORIENTED_EDGE ( 'NONE', *, *, #44338, .T. ) ;
#18996=CIRCLE ( 'NONE', #38636, 1.200000000000000178 ) ;
#19002=DIRECTION ( 'NONE',  ( -0.3127730236694430399, 0.9498278979187092519, 0.000000000000000000 ) ) ;
#19045=CARTESIAN_POINT ( 'NONE',  ( -2.109783507832979854, -6.917548591251819090, -19.00710507435085361 ) ) ;
#19046=CARTESIAN_POINT ( 'NONE',  ( 63.70438564670760684, -13.53232477329181727, -8.402906900370389565 ) ) ;
#19051=DIRECTION ( 'NONE',  ( -0.9908103287288504424, 0.1352586133457952533, 0.000000000000000000 ) ) ;
#19064=CARTESIAN_POINT ( 'NONE',  ( -13.36027627234077109, -3.983708254697501783, -18.97278025920458688 ) ) ;
#19088=CARTESIAN_POINT ( 'NONE',  ( 64.74132663541574573, -2.651366324200352231, -8.204703752599687760 ) ) ;
#19092=CARTESIAN_POINT ( 'NONE',  ( 66.98520468312386811, -0.07767352569349476876, -16.39321520033831447 ) ) ;
#19106=( BOUNDED_SURFACE ( )  B_SPLINE_SURFACE ( 3, 2, ( 
 ( #7955, #7728, #17551 ),
 ( #17772, #4532, #41952 ),
 ( #25295, #38500, #31667 ),
 ( #28493, #21640, #34846 ),
 ( #15029, #39422, #35761 ),
 ( #436, #4301, #21866 ),
 ( #32344, #32117, #35529 ),
 ( #3632, #42848, #42398 ),
 ( #10935, #1111, #11608 ),
 ( #28266, #11162, #31894 ),
 ( #42175, #25519, #31445 ),
 ( #38728, #38960, #214 ),
 ( #7500, #25067, #28044 ),
 ( #18223, #14127, #10716 ),
 ( #24617, #14804, #661 ),
 ( #28717, #24837, #21192 ) ),
 .UNSPECIFIED., .F., .F., .T. ) 
 B_SPLINE_SURFACE_WITH_KNOTS ( ( 4, 2, 2, 2, 2, 2, 2, 4 ),
 ( 3, 3 ),
 ( 0.000000000000000000, 0.001721917349777002610, 0.002582876024665504023, 0.003443834699554005219, 0.004304793374442506849, 0.005165752049331008046, 0.006026710724219509242, 0.006887669399108010439 ),
 ( 0.000000000000000000, 1.000000000000000000 ),
 .UNSPECIFIED. ) 
 GEOMETRIC_REPRESENTATION_ITEM ( )  RATIONAL_B_SPLINE_SURFACE ( (
 ( 1.000000000000000000, 0.7145271066604784727, 1.000000000000000000),
 ( 1.000000000000000000, 0.7222082868831993796, 1.000000000000000000),
 ( 1.000000000000000000, 0.7248468039590466594, 1.000000000000000000),
 ( 1.000000000000000000, 0.7198065179285114690, 1.000000000000000000),
 ( 1.000000000000000000, 0.7166470691620621114, 1.000000000000000000),
 ( 1.000000000000000000, 0.7075588989364935966, 1.000000000000000000),
 ( 1.000000000000000000, 0.7016239504775774183, 1.000000000000000000),
 ( 1.000000000000000000, 0.6870381831995848732, 1.000000000000000000),
 ( 1.000000000000000000, 0.6784604258937906307, 1.000000000000000000),
 ( 1.000000000000000000, 0.6592551312636351080, 1.000000000000000000),
 ( 1.000000000000000000, 0.6485902070625576554, 1.000000000000000000),
 ( 1.000000000000000000, 0.6253227720994979366, 1.000000000000000000),
 ( 1.000000000000000000, 0.6127475771026407170, 1.000000000000000000),
 ( 1.000000000000000000, 0.5864501210668879860, 1.000000000000000000),
 ( 1.000000000000000000, 0.5726586895731697879, 1.000000000000000000),
 ( 1.000000000000000000, 0.5583166281429867706, 1.000000000000000000) ) ) 
 REPRESENTATION_ITEM ( '' )  SURFACE ( )  );
#19115=AXIS2_PLACEMENT_3D ( 'NONE', #5973, #36974, #26743 ) ;
#19128=CARTESIAN_POINT ( 'NONE',  ( 61.94466824697356344, -46.76115691171892053, -16.39321520033831447 ) ) ;
#19134=EDGE_CURVE ( 'NONE', #11788, #26749, #43952, .T. ) ;
#19141=DIRECTION ( 'NONE',  ( -0.9986099732815398866, -0.05270788615228313989, 0.000000000000000000 ) ) ;
#19182=LINE ( 'NONE', #11896, #30356 ) ;
#19184=CIRCLE ( 'NONE', #20663, 0.5000000000000004441 ) ;
#19187=EDGE_CURVE ( 'NONE', #24192, #12356, #43135, .T. ) ;
#19188=CARTESIAN_POINT ( 'NONE',  ( 41.72636039845269096, -11.37347657059392070, -8.893215200338314474 ) ) ;
#19192=EDGE_CURVE ( 'NONE', #5970, #43660, #19866, .T. ) ;
#19209=CIRCLE ( 'NONE', #6083, 25.00000000000000355 ) ;
#19242=LINE ( 'NONE', #26081, #28473 ) ;
#19248=CIRCLE ( 'NONE', #14849, 4.999999999999998224 ) ;
#19277=CARTESIAN_POINT ( 'NONE',  ( 67.83464944830059551, -0.4399173918952799522, -10.39321520033831803 ) ) ;
#19279=CARTESIAN_POINT ( 'NONE',  ( 53.69308256885118169, -7.449060273445263114, -17.89321520033831447 ) ) ;
#19286=EDGE_CURVE ( 'NONE', #44000, #38238, #30129, .T. ) ;
#19292=DIRECTION ( 'NONE',  ( -0.9908103287288505534, 0.1352586133457950590, 0.000000000000000000 ) ) ;
#19295=CARTESIAN_POINT ( 'NONE',  ( -13.46025930250415925, -4.921265112563996347, -18.14637807345946996 ) ) ;
#19304=AXIS2_PLACEMENT_3D ( 'NONE', #37369, #45127, #34391 ) ;
#19321=CARTESIAN_POINT ( 'NONE',  ( 67.86702936097370298, -0.4719278425800559895, -16.39321520033831092 ) ) ;
#19326=CIRCLE ( 'NONE', #5481, 0.5000000000000004441 ) ;
#19341=CARTESIAN_POINT ( 'NONE',  ( 76.63408154409412987, 1.697290617957241565, -19.39321520033831447 ) ) ;
#19345=ORIENTED_EDGE ( 'NONE', *, *, #25993, .T. ) ;
#19352=VERTEX_POINT ( 'NONE', #19188 ) ;
#19368=ORIENTED_EDGE ( 'NONE', *, *, #35297, .T. ) ;
#19397=( GEOMETRIC_REPRESENTATION_CONTEXT ( 3 ) GLOBAL_UNCERTAINTY_ASSIGNED_CONTEXT ( ( #22380 ) ) GLOBAL_UNIT_ASSIGNED_CONTEXT ( ( #29392, #32127, #22104 ) ) REPRESENTATION_CONTEXT ( 'NONE', 'WORKASPACE' ) );
#19398=AXIS2_PLACEMENT_3D ( 'NONE', #1203, #43379, #32868 ) ;
#19411=EDGE_LOOP ( 'NONE', ( #34647, #5699, #17512, #6573 ) ) ;
#19456=CARTESIAN_POINT ( 'NONE',  ( -2.417516882670096123, -7.009994832972470391, -7.554101583258010955 ) ) ;
#19476=EDGE_CURVE ( 'NONE', #4486, #31639, #8276, .T. ) ;
#19487=CARTESIAN_POINT ( 'NONE',  ( 71.31713442278434911, 2.423123680056909368, -16.18610841915176479 ) ) ;
#19491=EDGE_CURVE ( 'NONE', #41326, #19352, #41963, .T. ) ;
#19498=CARTESIAN_POINT ( 'NONE',  ( 67.79187456311957760, -0.4014585417718678495, -10.39321520033831447 ) ) ;
#19503=ORIENTED_EDGE ( 'NONE', *, *, #8947, .F. ) ;
#19544=CARTESIAN_POINT ( 'NONE',  ( 67.52555172610438206, -0.2286232172799360363, -16.39321520033831803 ) ) ;
#19555=ADVANCED_FACE ( 'NONE', ( #27160 ), #44724, .T. ) ;
#19558=CARTESIAN_POINT ( 'NONE',  ( 3.060777270043529619, -5.064559853354640317, -17.89321520033831447 ) ) ;
#19568=EDGE_LOOP ( 'NONE', ( #31183, #43520, #44568, #17580 ) ) ;
#19618=DIRECTION ( 'NONE',  ( -0.9908103287288503314, 0.1352586133457956419, 0.000000000000000000 ) ) ;
#19625=EDGE_LOOP ( 'NONE', ( #26834, #3242, #24528, #23051 ) ) ;
#19651=ORIENTED_EDGE ( 'NONE', *, *, #33363, .T. ) ;
#19679=CARTESIAN_POINT ( 'NONE',  ( -2.848861189601162192, -7.139067047498250496, -7.411210244931162094 ) ) ;
#19719=CARTESIAN_POINT ( 'NONE',  ( 65.98944182936091352, -0.1558845086392504908, -10.39321520033831447 ) ) ;
#19728=ADVANCED_FACE ( 'NONE', ( #3645 ), #31458, .F. ) ;
#19736=CIRCLE ( 'NONE', #26278, 1.499999999999999334 ) ;
#19754=ORIENTED_EDGE ( 'NONE', *, *, #19789, .T. ) ;
#19769=AXIS2_PLACEMENT_3D ( 'NONE', #27011, #30656, #23832 ) ;
#19771=CARTESIAN_POINT ( 'NONE',  ( 75.95778847736514194, -3.256761025687008537, -16.39321520033831447 ) ) ;
#19789=EDGE_CURVE ( 'NONE', #19947, #873, #27164, .T. ) ;
#19804=ORIENTED_EDGE ( 'NONE', *, *, #9439, .F. ) ;
#19832=CARTESIAN_POINT ( 'NONE',  ( 68.56885555382550024, -20.41671115022304406, -19.39321520033831447 ) ) ;
#19866=LINE ( 'NONE', #22601, #23486 ) ;
#19882=ORIENTED_EDGE ( 'NONE', *, *, #40713, .T. ) ;
#19897=CIRCLE ( 'NONE', #3868, 6.500000000000000888 ) ;
#19898=DIRECTION ( 'NONE',  ( -0.9908103287288504424, 0.1352586133457950590, 0.000000000000000000 ) ) ;
#19911=FACE_OUTER_BOUND ( 'NONE', #7806, .T. ) ;
#19916=CARTESIAN_POINT ( 'NONE',  ( -2.700297285702341732, -7.094665554431733412, -7.444873403169903092 ) ) ;
#19947=VERTEX_POINT ( 'NONE', #29843 ) ;
#19951=CARTESIAN_POINT ( 'NONE',  ( 67.05591816083881440, -0.08547223048874456885, -10.39321520033831447 ) ) ;
#19965=LINE ( 'NONE', #23163, #1145 ) ;
#19971=DIRECTION ( 'NONE',  ( 0.000000000000000000, 0.000000000000000000, -1.000000000000000000 ) ) ;
#20016=EDGE_CURVE ( 'NONE', #26194, #24134, #39659, .T. ) ;
#20037=ORIENTED_EDGE ( 'NONE', *, *, #41247, .T. ) ;
#20042=DIRECTION ( 'NONE',  ( 0.9908103287288505534, -0.1352586133457944206, 0.000000000000000000 ) ) ;
#20045=EDGE_CURVE ( 'NONE', #22059, #16290, #32214, .T. ) ;
#20057=ORIENTED_EDGE ( 'NONE', *, *, #44280, .T. ) ;
#20062=CARTESIAN_POINT ( 'NONE',  ( 66.58723489636778936, -20.14619392353143112, -10.89321520033831447 ) ) ;
#20080=LINE ( 'NONE', #9360, #13850 ) ;
#20098=CARTESIAN_POINT ( 'NONE',  ( 69.69189222815028018, -41.76310523276638520, -7.393215200338315363 ) ) ;
#20101=ORIENTED_EDGE ( 'NONE', *, *, #6114, .F. ) ;
#20112=VERTEX_POINT ( 'NONE', #40565 ) ;
#20117=DIRECTION ( 'NONE',  ( 0.7962509850245451659, 0.6049664196031392382, 0.000000000000000000 ) ) ;
#20143=CARTESIAN_POINT ( 'NONE',  ( 60.06931813437628875, -14.72076136720887085, -18.18301750815651374 ) ) ;
#20147=FACE_OUTER_BOUND ( 'NONE', #15077, .T. ) ;
#20149=DIRECTION ( 'NONE',  ( -0.9908103287288504424, 0.1352586133457950590, 0.000000000000000000 ) ) ;
#20169=VECTOR ( 'NONE', #23935, 1000.000000000000000 ) ;
#20199=DIRECTION ( 'NONE',  ( 0.000000000000000000, 0.000000000000000000, -1.000000000000000000 ) ) ;
#20201=CARTESIAN_POINT ( 'NONE',  ( 61.05647571779960003, -46.63990697477660063, -12.39321520033831447 ) ) ;
#20226=CIRCLE ( 'NONE', #30412, 2.999999999999996003 ) ;
#20241=CARTESIAN_POINT ( 'NONE',  ( 41.72636039845269096, -11.37347657059392070, -10.39321520033831625 ) ) ;
#20277=ADVANCED_FACE ( 'NONE', ( #13867 ), #23556, .T. ) ;
#20287=DIRECTION ( 'NONE',  ( -0.9908103287288504424, 0.1352586133457951423, 0.000000000000000000 ) ) ;
#20308=ADVANCED_FACE ( 'NONE', ( #9549 ), #37351, .T. ) ;
#20309=FACE_OUTER_BOUND ( 'NONE', #13858, .T. ) ;
#20334=EDGE_CURVE ( 'NONE', #4744, #31560, #19897, .T. ) ;
#20352=DIRECTION ( 'NONE',  ( 0.9908103287288504424, -0.1352586133457950035, 0.000000000000000000 ) ) ;
#20365=LINE ( 'NONE', #27205, #3756 ) ;
#20383=ORIENTED_EDGE ( 'NONE', *, *, #15305, .T. ) ;
#20384=EDGE_CURVE ( 'NONE', #23226, #18085, #44132, .T. ) ;
#20416=ORIENTED_EDGE ( 'NONE', *, *, #29573, .T. ) ;
#20436=EDGE_CURVE ( 'NONE', #42783, #3386, #31824, .T. ) ;
#20437=EDGE_LOOP ( 'NONE', ( #698, #1376, #12903, #41529 ) ) ;
#20477=AXIS2_PLACEMENT_3D ( 'NONE', #36105, #32897, #26309 ) ;
#20479=DIRECTION ( 'NONE',  ( 0.1352586133457957807, 0.9908103287288503314, 0.000000000000000000 ) ) ;
#20502=DIRECTION ( 'NONE',  ( -0.9063289528979890930, -0.4225728684367167087, 0.000000000000000000 ) ) ;
#20507=ORIENTED_EDGE ( 'NONE', *, *, #41247, .F. ) ;
#20530=ORIENTED_EDGE ( 'NONE', *, *, #25373, .T. ) ;
#20554=CARTESIAN_POINT ( 'NONE',  ( 61.46741937898128327, -12.47125186204822178, -9.654607599614944746 ) ) ;
#20565=CARTESIAN_POINT ( 'NONE',  ( 59.92022724782403742, -14.76985616374063426, -18.18981531286807041 ) ) ;
#20570=FACE_OUTER_BOUND ( 'NONE', #45080, .T. ) ;
#20625=ADVANCED_FACE ( 'NONE', ( #23050 ), #26478, .F. ) ;
#20652=DIRECTION ( 'NONE',  ( 0.1352586133457954198, 0.9908103287288503314, 0.000000000000000000 ) ) ;
#20663=AXIS2_PLACEMENT_3D ( 'NONE', #7546, #34072, #14851 ) ;
#20669=CIRCLE ( 'NONE', #37375, 1.500000000000000000 ) ;
#20675=CARTESIAN_POINT ( 'NONE',  ( 65.53695226829334786, -0.2718670794236524024, -8.259322725476325289 ) ) ;
#20680=LINE ( 'NONE', #42096, #38200 ) ;
#20681=CARTESIAN_POINT ( 'NONE',  ( 59.44377208703740223, -12.82110557137145967, -17.39288367676203606 ) ) ;
#20691=CARTESIAN_POINT ( 'NONE',  ( 71.31713442278437753, 2.423123680056944007, -10.89321520033831447 ) ) ;
#20702=DIRECTION ( 'NONE',  ( 0.000000000000000000, 0.000000000000000000, -1.000000000000000000 ) ) ;
#20715=DIRECTION ( 'NONE',  ( 0.000000000000000000, 0.000000000000000000, 1.000000000000000000 ) ) ;
#20728=CARTESIAN_POINT ( 'NONE',  ( -13.90346622911622276, -4.337920416975670435, -8.893215200338337567 ) ) ;
#20735=TOROIDAL_SURFACE ( 'NONE', #34545, 4.500000000000000000, 1.500000000000000000 ) ;
#20759=EDGE_LOOP ( 'NONE', ( #1211, #8928, #15782, #21068 ) ) ;
#20769=AXIS2_PLACEMENT_3D ( 'NONE', #17149, #2773, #44510 ) ;
#20781=VERTEX_POINT ( 'NONE', #33508 ) ;
#20788=CARTESIAN_POINT ( 'NONE',  ( 31.16203868753470019, 11.28474725185576055, -8.893215200338314474 ) ) ;
#20896=TOROIDAL_SURFACE ( 'NONE', #18707, 12.50000000000000000, 1.500000000000000000 ) ;
#20901=CARTESIAN_POINT ( 'NONE',  ( 61.17398009194395314, -12.48488768724098108, -17.20141017814964357 ) ) ;
#20906=FACE_OUTER_BOUND ( 'NONE', #35785, .T. ) ;
#20938=B_SPLINE_CURVE_WITH_KNOTS ( 'NONE', 3,
 ( #799, #42313, #14942, #7410, #36119, #14717, #28403, #35898, #31808, #11072, #18585, #38871, #21330, #4664 ),
 .UNSPECIFIED., .F., .F.,
 ( 4, 2, 2, 2, 2, 2, 4 ),
 ( 0.006010506521692418960, 0.007331959427853154687, 0.007992685880933507805, 0.008653412334013860924, 0.009314138787094194960, 0.009974865240174530731, 0.01129631814633520054 ),
 .UNSPECIFIED. ) ;
#20944=LINE ( 'NONE', #24587, #28573 ) ;
#20946=ORIENTED_EDGE ( 'NONE', *, *, #11364, .F. ) ;
#20950=CARTESIAN_POINT ( 'NONE',  ( 27.57768543387103222, -14.97172645945875935, -8.893215200338314474 ) ) ;
#20952=FACE_OUTER_BOUND ( 'NONE', #32196, .T. ) ;
#20961=DIRECTION ( 'NONE',  ( -0.9498278979187093629, -0.3127730236694430954, 0.000000000000000000 ) ) ;
#20963=ORIENTED_EDGE ( 'NONE', *, *, #24911, .F. ) ;
#21004=DIRECTION ( 'NONE',  ( 0.1352586133457950590, 0.9908103287288504424, 0.000000000000000000 ) ) ;
#21006=DIRECTION ( 'NONE',  ( 0.9063289528979890930, 0.4225728684367167087, 0.000000000000000000 ) ) ;
#21011=CARTESIAN_POINT ( 'NONE',  ( 64.57998409241588433, -15.42822026892965326, -16.02015606411926996 ) ) ;
#21054=CARTESIAN_POINT ( 'NONE',  ( 75.95778847736514194, -3.256761025687008537, -7.147228641687434880 ) ) ;
#21068=ORIENTED_EDGE ( 'NONE', *, *, #18422, .F. ) ;
#21076=CARTESIAN_POINT ( 'NONE',  ( 60.49017502987772588, -14.58217554126443893, -18.15922316508111933 ) ) ;
#21098=CARTESIAN_POINT ( 'NONE',  ( 42.36021970110777346, -12.73296999994090761, -19.39321520033831447 ) ) ;
#21100=CARTESIAN_POINT ( 'NONE',  ( 59.90552009294155766, -2.897503654462286971, -7.393215200338319804 ) ) ;
#21101=CYLINDRICAL_SURFACE ( 'NONE', #8433, 4.999999999999997335 ) ;
#21102=EDGE_CURVE ( 'NONE', #24192, #35546, #32954, .T. ) ;
#21110=CARTESIAN_POINT ( 'NONE',  ( 59.90552009294157898, -2.897503654462289191, -8.893215200338314474 ) ) ;
#21111=B_SPLINE_CURVE_WITH_KNOTS ( 'NONE', 3,
 ( #21721, #7812, #14881, #29679, #26038, #1191 ),
 .UNSPECIFIED., .F., .F.,
 ( 4, 2, 4 ),
 ( 0.001955951169366054645, 0.002520422424572374680, 0.003084893679778694716 ),
 .UNSPECIFIED. ) ;
#21115=CARTESIAN_POINT ( 'NONE',  ( 76.36356431740252049, -0.2843300395004543235, -12.39321520033831447 ) ) ;
#21143=ADVANCED_FACE ( 'NONE', ( #22488, #25695 ), #3854, .T. ) ;
#21184=DIRECTION ( 'NONE',  ( -0.05270788615228318846, 0.9986099732815399976, 2.696077241641140828E-16 ) ) ;
#21192=CARTESIAN_POINT ( 'NONE',  ( 64.78873258728907558, -15.59143358259173873, -15.46696664105744290 ) ) ;
#21225=CARTESIAN_POINT ( 'NONE',  ( 59.41811746136757222, -12.82955349636864639, -9.393325708960333031 ) ) ;
#21234=( BOUNDED_SURFACE ( )  B_SPLINE_SURFACE ( 3, 2, ( 
 ( #23169, #26360, #43468 ),
 ( #12008, #33394, #8801 ),
 ( #29101, #1285, #43917 ),
 ( #39595, #25910, #12459 ),
 ( #19295, #36376, #11781 ),
 ( #9259, #39815, #19064 ),
 ( #36824, #2168, #15197 ),
 ( #22705, #22260, #5378 ),
 ( #5593, #5147, #30001 ),
 ( #12686, #5819, #37048 ),
 ( #26585, #33173, #1950 ),
 ( #15876, #29773, #43684 ) ),
 .UNSPECIFIED., .F., .F., .F. ) 
 B_SPLINE_SURFACE_WITH_KNOTS ( ( 4, 2, 2, 2, 2, 4 ),
 ( 3, 3 ),
 ( 0.001037087982888927054, 0.001174868562012537990, 0.001312649141136149143, 0.001381539430697954719, 0.001450429720259760295, 0.001588210299383371448 ),
 ( 0.000000000000000000, 1.000000000000000000 ),
 .UNSPECIFIED. ) 
 GEOMETRIC_REPRESENTATION_ITEM ( )  RATIONAL_B_SPLINE_SURFACE ( (
 ( 1.000000000000000000, 0.7071067811865475727, 1.000000000000000000),
 ( 1.000000000000000000, 0.7345423267586178584, 1.000000000000000000),
 ( 1.000000000000000000, 0.7596204909257884275, 1.000000000000000000),
 ( 1.000000000000000000, 0.8061747443791169587, 1.000000000000000000),
 ( 1.000000000000000000, 0.8273618726001445989, 1.000000000000000000),
 ( 1.000000000000000000, 0.8547411548254547631, 1.000000000000000000),
 ( 1.000000000000000000, 0.8633031996701927557, 1.000000000000000000),
 ( 1.000000000000000000, 0.8784466432148445580, 1.000000000000000000),
 ( 1.000000000000000000, 0.8850520986738202867, 1.000000000000000000),
 ( 1.000000000000000000, 0.9017204459549897910, 1.000000000000000000),
 ( 1.000000000000000000, 0.9078805346385753205, 1.000000000000000000),
 ( 1.000000000000000000, 0.9079001203735741488, 1.000000000000000000) ) ) 
 REPRESENTATION_ITEM ( '' )  SURFACE ( )  );
#21237=ORIENTED_EDGE ( 'NONE', *, *, #16124, .T. ) ;
#21288=VECTOR ( 'NONE', #40850, 1000.000000000000000 ) ;
#21295=ORIENTED_EDGE ( 'NONE', *, *, #25124, .F. ) ;
#21310=CARTESIAN_POINT ( 'NONE',  ( 65.23579839261728353, -13.46795819349411616, -11.98898727572936451 ) ) ;
#21323=EDGE_LOOP ( 'NONE', ( #2665, #19804, #29725, #29503 ) ) ;
#21330=CARTESIAN_POINT ( 'NONE',  ( 60.49017502987946671, -14.58217554126384563, -8.627207235595617973 ) ) ;
#21333=CIRCLE ( 'NONE', #27176, 0.5000000000000044409 ) ;
#21337=CARTESIAN_POINT ( 'NONE',  ( 60.46773714784079345, -12.56592564749740148, -17.32492254961432820 ) ) ;
#21393=EDGE_CURVE ( 'NONE', #12130, #8541, #5339, .T. ) ;
#21405=ORIENTED_EDGE ( 'NONE', *, *, #13329, .F. ) ;
#21415=CARTESIAN_POINT ( 'NONE',  ( 59.24641515291911986, -13.72835195454734247, -19.39321520033831447 ) ) ;
#21428=DIRECTION ( 'NONE',  ( 0.9908103287288504424, -0.1352586133457950590, 0.000000000000000000 ) ) ;
#21433=MANIFOLD_SOLID_BREP ( 'NONE', #1747 ) ;
#21443=AXIS2_PLACEMENT_3D ( 'NONE', #28198, #38653, #24989 ) ;
#21460=ORIENTED_EDGE ( 'NONE', *, *, #42866, .T. ) ;
#21480=CARTESIAN_POINT ( 'NONE',  ( -6.962123463324038752, -11.49046785505262669, -8.593215200338315540 ) ) ;
#21488=AXIS2_PLACEMENT_3D ( 'NONE', #9012, #43216, #22682 ) ;
#21494=EDGE_CURVE ( 'NONE', #23361, #19352, #19209, .T. ) ;
#21505=LINE ( 'NONE', #305, #31757 ) ;
#21510=ADVANCED_FACE ( 'NONE', ( #1571 ), #24432, .T. ) ;
#21527=CARTESIAN_POINT ( 'NONE',  ( 0.04488520489200759078, -6.166763362545027327, -19.39321520033831447 ) ) ;
#21533=CARTESIAN_POINT ( 'NONE',  ( 64.80575110624921820, -13.22907879418145249, -11.52632176784967655 ) ) ;
#21549=AXIS2_PLACEMENT_3D ( 'NONE', #11026, #24926, #3718 ) ;
#21551=CIRCLE ( 'NONE', #29563, 10.00000000000000000 ) ;
#21562=CARTESIAN_POINT ( 'NONE',  ( 60.83824608292380987, -12.51476863122120520, -17.26777189981386229 ) ) ;
#21569=CARTESIAN_POINT ( 'NONE',  ( 64.51132457273422460, -13.77492255257581277, -8.859678336860978831 ) ) ;
#21580=CARTESIAN_POINT ( 'NONE',  ( -3.429934629567074733, -4.841764211284793618, -7.393215200338315363 ) ) ;
#21612=ORIENTED_EDGE ( 'NONE', *, *, #12672, .F. ) ;
#21614=CARTESIAN_POINT ( 'NONE',  ( -13.55413964183373743, -3.899881072927508185, -8.039791994638363803 ) ) ;
#21619=DIRECTION ( 'NONE',  ( -0.9908103287288504424, 0.1352586133457950590, 0.000000000000000000 ) ) ;
#21640=CARTESIAN_POINT ( 'NONE',  ( 61.95510581920947146, -14.46403044595587595, -19.00299887994344061 ) ) ;
#21649=DIRECTION ( 'NONE',  ( 0.000000000000000000, 0.000000000000000000, 1.000000000000000000 ) ) ;
#21665=DIRECTION ( 'NONE',  ( -0.000000000000000000, -0.000000000000000000, 1.000000000000000000 ) ) ;
#21698=DIRECTION ( 'NONE',  ( 0.000000000000000000, 0.000000000000000000, 1.000000000000000000 ) ) ;
#21714=ORIENTED_EDGE ( 'NONE', *, *, #10964, .T. ) ;
#21721=CARTESIAN_POINT ( 'NONE',  ( 65.41257106814472877, -15.47412461924279725, -10.39321520033831625 ) ) ;
#21734=CARTESIAN_POINT ( 'NONE',  ( 69.69189222815028018, -41.76310523276638520, -19.39321520033831447 ) ) ;
#21753=LINE ( 'NONE', #31558, #5307 ) ;
#21760=CARTESIAN_POINT ( 'NONE',  ( 63.53803937314328465, -12.73310566472691185, -10.53259732128069537 ) ) ;
#21786=CARTESIAN_POINT ( 'NONE',  ( -13.56828337869051104, -4.779084862086333985, -17.89321520033831447 ) ) ;
#21788=CARTESIAN_POINT ( 'NONE',  ( 64.17925045615415058, -12.94885914896418377, -15.80747231013753940 ) ) ;
#21789=CARTESIAN_POINT ( 'NONE',  ( -12.55610316477683241, -4.307149106694457608, -7.393215200338315363 ) ) ;
#21792=CARTESIAN_POINT ( 'NONE',  ( 42.36021970110777346, -12.73296999994090584, -17.89321520033831447 ) ) ;
#21811=DIRECTION ( 'NONE',  ( -0.1352586133457954198, -0.9908103287288503314, 0.000000000000000000 ) ) ;
#21835=ORIENTED_EDGE ( 'NONE', *, *, #21934, .T. ) ;
#21863=CARTESIAN_POINT ( 'NONE',  ( 2.181596283295915484, -11.50482699009217669, -17.89321520033831447 ) ) ;
#21866=CARTESIAN_POINT ( 'NONE',  ( 62.31167178596560774, -14.51130963312466626, -17.61767033193244103 ) ) ;
#21878=FACE_OUTER_BOUND ( 'NONE', #37850, .T. ) ;
#21880=ORIENTED_EDGE ( 'NONE', *, *, #25317, .T. ) ;
#21883=CARTESIAN_POINT ( 'NONE',  ( 66.83265463627490988, 0.3322498524448982415, -17.83539872533922122 ) ) ;
#21920=CARTESIAN_POINT ( 'NONE',  ( 61.93156847455979630, -13.30602482174417034, -19.05359815343103236 ) ) ;
#21929=CIRCLE ( 'NONE', #8101, 5.000000000000000000 ) ;
#21933=ORIENTED_EDGE ( 'NONE', *, *, #17126, .T. ) ;
#21934=EDGE_CURVE ( 'NONE', #32179, #38238, #20669, .T. ) ;
#21952=CARTESIAN_POINT ( 'NONE',  ( 74.43213512091445239, -36.61236768192972590, -7.393215200338315363 ) ) ;
#21977=CARTESIAN_POINT ( 'NONE',  ( 62.36331481589586900, -14.51968798477179412, -17.59173035813085662 ) ) ;
#21979=EDGE_LOOP ( 'NONE', ( #44332, #31897, #31005, #15218, #24914 ) ) ;
#21991=ORIENTED_EDGE ( 'NONE', *, *, #20384, .F. ) ;
#22007=DIRECTION ( 'NONE',  ( -0.9908103287288504424, 0.1352586133457951423, 0.000000000000000000 ) ) ;
#22012=CARTESIAN_POINT ( 'NONE',  ( 35.90261398037149121, 14.17005867477686820, -18.19321520033831519 ) ) ;
#22016=AXIS2_PLACEMENT_3D ( 'NONE', #5227, #43998, #19141 ) ;
#22018=CARTESIAN_POINT ( 'NONE',  ( 63.48716809568579578, -14.78506867088062471, -8.380858988663437259 ) ) ;
#22059=VERTEX_POINT ( 'NONE', #10020 ) ;
#22065=CARTESIAN_POINT ( 'NONE',  ( -13.40759878756898260, -4.990576376016446325, -7.482946478807211754 ) ) ;
#22075=AXIS2_PLACEMENT_3D ( 'NONE', #6799, #3370, #17289 ) ;
#22083=CARTESIAN_POINT ( 'NONE',  ( 59.90552009294157898, -2.897503654462289191, -17.89321520033831447 ) ) ;
#22104=( NAMED_UNIT ( * ) SI_UNIT ( $, .STERADIAN. ) SOLID_ANGLE_UNIT ( ) );
#22107=ORIENTED_EDGE ( 'NONE', *, *, #41910, .F. ) ;
#22153=CARTESIAN_POINT ( 'NONE',  ( -1.145390592550938669, -14.88589425535891841, -19.39321520033831447 ) ) ;
#22228=DIRECTION ( 'NONE',  ( 0.000000000000000000, 0.000000000000000000, 1.000000000000000000 ) ) ;
#22231=CARTESIAN_POINT ( 'NONE',  ( 64.59716620846640467, -13.12735690504239017, -15.45707635952990344 ) ) ;
#22237=CARTESIAN_POINT ( 'NONE',  ( -1.813282010071980421, -6.828405667812914359, -18.61931990332739062 ) ) ;
#22238=CARTESIAN_POINT ( 'NONE',  ( 65.01231714173856346, -15.66127537904516132, -9.355441156750886833 ) ) ;
#22253=TOROIDAL_SURFACE ( 'NONE', #30981, 26.50000000000000000, 1.500000000000000000 ) ;
#22260=CARTESIAN_POINT ( 'NONE',  ( -13.82150966199706588, -4.445790862645441877, -18.50085597516207514 ) ) ;
#22287=ORIENTED_EDGE ( 'NONE', *, *, #35051, .T. ) ;
#22289=CARTESIAN_POINT ( 'NONE',  ( 67.69801799180082469, -1.521560346498090022, -9.966191704370915616 ) ) ;
#22303=DIRECTION ( 'NONE',  ( 0.000000000000000000, 0.000000000000000000, -1.000000000000000000 ) ) ;
#22319=CARTESIAN_POINT ( 'NONE',  ( 68.56885555382550024, -20.41671115022302274, -19.39321520033831447 ) ) ;
#22345=CARTESIAN_POINT ( 'NONE',  ( 75.95778847736514194, -3.256761025687008537, -14.39321520033831625 ) ) ;
#22357=VECTOR ( 'NONE', #8828, 1000.000000000000000 ) ;
#22360=CARTESIAN_POINT ( 'NONE',  ( 75.95778847736514194, -3.256761025687008537, -10.89321520033831447 ) ) ;
#22378=CARTESIAN_POINT ( 'NONE',  ( 46.84966980880212617, -19.07391775237791620, -19.39321520033831447 ) ) ;
#22380=UNCERTAINTY_MEASURE_WITH_UNIT (LENGTH_MEASURE( 1.000000000000000082E-05 ), #29392, 'distance_accuracy_value', 'NONE');
#22385=EDGE_CURVE ( 'NONE', #16955, #22059, #35724, .T. ) ;
#22424=CARTESIAN_POINT ( 'NONE',  ( 46.22412376146323965, -17.17426195654049437, -19.39321520033831447 ) ) ;
#22426=ORIENTED_EDGE ( 'NONE', *, *, #23688, .T. ) ;
#22433=LINE ( 'NONE', #32683, #41578 ) ;
#22464=CARTESIAN_POINT ( 'NONE',  ( 66.21645592411296377, -14.64013927798640502, -10.27431999848409028 ) ) ;
#22468=DIRECTION ( 'NONE',  ( -0.1352586133457950590, -0.9908103287288504424, 0.000000000000000000 ) ) ;
#22488=FACE_BOUND ( 'NONE', #788, .T. ) ;
#22502=ORIENTED_EDGE ( 'NONE', *, *, #29788, .F. ) ;
#22508=CARTESIAN_POINT ( 'NONE',  ( 64.97240540738540915, -2.563123825349247209, -8.300243185318032957 ) ) ;
#22558=ORIENTED_EDGE ( 'NONE', *, *, #36467, .F. ) ;
#22586=ORIENTED_EDGE ( 'NONE', *, *, #26511, .F. ) ;
#22595=ORIENTED_EDGE ( 'NONE', *, *, #33629, .T. ) ;
#22601=CARTESIAN_POINT ( 'NONE',  ( 46.84966980880212617, -19.07391775237791620, -19.39321520033831447 ) ) ;
#22623=DIRECTION ( 'NONE',  ( -0.9908103287288505534, 0.1352586133457950313, 0.000000000000000000 ) ) ;
#22631=ORIENTED_EDGE ( 'NONE', *, *, #19192, .T. ) ;
#22650=CARTESIAN_POINT ( 'NONE',  ( -2.081610404626085042, -6.909071579789481277, -7.809159120385307240 ) ) ;
#22668=VECTOR ( 'NONE', #11661, 1000.000000000000114 ) ;
#22680=CARTESIAN_POINT ( 'NONE',  ( 64.49285160086900248, -13.07967021556595100, -15.54970782244410010 ) ) ;
#22682=DIRECTION ( 'NONE',  ( 0.000000000000000000, 1.387778780781444413E-14, -1.000000000000000000 ) ) ;
#22686=CARTESIAN_POINT ( 'NONE',  ( 65.94404352776260225, -0.1671492176496161552, -10.39321520033831625 ) ) ;
#22687=CIRCLE ( 'NONE', #19769, 0.5000000000000004441 ) ;
#22688=CARTESIAN_POINT ( 'NONE',  ( -2.434349165179547914, -7.015039675730945667, -19.23631625773906961 ) ) ;
#22703=CARTESIAN_POINT ( 'NONE',  ( -13.50764450192301602, -4.858897168674483069, -8.690106464020692201 ) ) ;
#22705=CARTESIAN_POINT ( 'NONE',  ( -13.52723683684260614, -4.833109925824063957, -18.06246285863358736 ) ) ;
#22753=LINE ( 'NONE', #12734, #34969 ) ;
#22762=VERTEX_POINT ( 'NONE', #21110 ) ;
#22763=TOROIDAL_SURFACE ( 'NONE', #12560, 33.80000000000000426, 1.199999999999999956 ) ;
#22835=EDGE_LOOP ( 'NONE', ( #16299, #44284, #9411, #9086 ) ) ;
#22839=EDGE_CURVE ( 'NONE', #15605, #35231, #32864, .T. ) ;
#22865=ORIENTED_EDGE ( 'NONE', *, *, #19192, .F. ) ;
#22880=DIRECTION ( 'NONE',  ( 0.000000000000000000, 0.000000000000000000, 1.000000000000000000 ) ) ;
#22914=CARTESIAN_POINT ( 'NONE',  ( 66.95179978577000668, -0.07398856205378337436, -10.39321520033831447 ) ) ;
#22915=LINE ( 'NONE', #32489, #12949 ) ;
#22928=CARTESIAN_POINT ( 'NONE',  ( 59.24641515291911986, -13.72835195454734247, -8.593215200338315540 ) ) ;
#22938=ORIENTED_EDGE ( 'NONE', *, *, #18920, .T. ) ;
#22941=AXIS2_PLACEMENT_3D ( 'NONE', #42650, #14606, #38992 ) ;
#22961=CARTESIAN_POINT ( 'NONE',  ( 67.42128206111212307, -0.1796520177129405649, -16.39321520033831447 ) ) ;
#22995=ORIENTED_EDGE ( 'NONE', *, *, #5061, .F. ) ;
#23047=CIRCLE ( 'NONE', #15044, 1.499999999999999556 ) ;
#23050=FACE_OUTER_BOUND ( 'NONE', #8787, .T. ) ;
#23051=ORIENTED_EDGE ( 'NONE', *, *, #30594, .F. ) ;
#23073=ORIENTED_EDGE ( 'NONE', *, *, #12309, .T. ) ;
#23076=CARTESIAN_POINT ( 'NONE',  ( 65.83173732663925648, -15.38336477915846245, -16.39321520033830737 ) ) ;
#23107=CARTESIAN_POINT ( 'NONE',  ( 64.65782898596719974, -2.683267933343334910, -18.61496147612403362 ) ) ;
#23108=FACE_OUTER_BOUND ( 'NONE', #13024, .T. ) ;
#23112=CARTESIAN_POINT ( 'NONE',  ( -2.063229709340284046, -6.903538917046990520, -7.827879352907993749 ) ) ;
#23122=ORIENTED_EDGE ( 'NONE', *, *, #28259, .T. ) ;
#23133=AXIS2_PLACEMENT_3D ( 'NONE', #42724, #8062, #15801 ) ;
#23149=CARTESIAN_POINT ( 'NONE',  ( 68.14371629974728251, -1.351251493923715685, -10.39321520033831625 ) ) ;
#23150=FACE_BOUND ( 'NONE', #8121, .T. ) ;
#23163=CARTESIAN_POINT ( 'NONE',  ( -7.917624645353497748, -12.21642755857638818, -8.593215200338315540 ) ) ;
#23169=CARTESIAN_POINT ( 'NONE',  ( -13.32377113153209791, -5.100909530930219482, -18.19321520033831874 ) ) ;
#23226=VERTEX_POINT ( 'NONE', #7149 ) ;
#23228=ORIENTED_EDGE ( 'NONE', *, *, #1314, .T. ) ;
#23289=AXIS2_PLACEMENT_3D ( 'NONE', #3979, #18575, #18355 ) ;
#23298=ORIENTED_EDGE ( 'NONE', *, *, #3869, .T. ) ;
#23303=LINE ( 'NONE', #37186, #9807 ) ;
#23328=CARTESIAN_POINT ( 'NONE',  ( 65.37779407113983154, -2.408155782755655672, -18.33092689054683078 ) ) ;
#23353=AXIS2_PLACEMENT_3D ( 'NONE', #4855, #1213, #11707 ) ;
#23361=VERTEX_POINT ( 'NONE', #14673 ) ;
#23362=CARTESIAN_POINT ( 'NONE',  ( 59.75121349346655109, -13.58877957849837870, -7.404803486908546617 ) ) ;
#23366=CIRCLE ( 'NONE', #7343, 4.999999999999998224 ) ;
#23375=CARTESIAN_POINT ( 'NONE',  ( 67.82132387878262136, -0.4275346869931948013, -10.39321520033832158 ) ) ;
#23377=CYLINDRICAL_SURFACE ( 'NONE', #24378, 1.499999999999999556 ) ;
#23403=ADVANCED_FACE ( 'NONE', ( #11931 ), #5070, .T. ) ;
#23426=EDGE_CURVE ( 'NONE', #33232, #28936, #18320, .T. ) ;
#23481=EDGE_CURVE ( 'NONE', #43660, #10084, #33460, .T. ) ;
#23486=VECTOR ( 'NONE', #12806, 1000.000000000000000 ) ;
#23552=DIRECTION ( 'NONE',  ( 0.000000000000000000, 0.000000000000000000, 1.000000000000000000 ) ) ;
#23556=TOROIDAL_SURFACE ( 'NONE', #35162, 5.500000000000000000, 0.5000000000000000000 ) ;
#23567=CARTESIAN_POINT ( 'NONE',  ( 59.41474631770697101, -13.68180984308303216, -19.39321520033831803 ) ) ;
#23597=CYLINDRICAL_SURFACE ( 'NONE', #35359, 1.499999999999998002 ) ;
#23624=B_SPLINE_CURVE_WITH_KNOTS ( 'NONE', 3,
 ( #1488, #26349, #40257, #15410, #33384, #29990, #43456, #40488, #29540, #2156 ),
 .UNSPECIFIED., .F., .F.,
 ( 4, 2, 2, 2, 4 ),
 ( 3.469446951953614189E-18, 0.0003217971434675209806, 0.0006435942869350384917, 0.0009653914304025559487, 0.001287188573870073514 ),
 .UNSPECIFIED. ) ;
#23633=VERTEX_POINT ( 'NONE', #11257 ) ;
#23652=CARTESIAN_POINT ( 'NONE',  ( 59.24641515291911986, -13.72835195454734247, -19.39321520033831447 ) ) ;
#23654=DIRECTION ( 'NONE',  ( 0.000000000000000000, 0.000000000000000000, 1.000000000000000000 ) ) ;
#23655=ADVANCED_FACE ( 'NONE', ( #39063 ), #36079, .F. ) ;
#23659=LINE ( 'NONE', #38000, #25296 ) ;
#23670=EDGE_CURVE ( 'NONE', #15605, #31742, #15124, .T. ) ;
#23680=ORIENTED_EDGE ( 'NONE', *, *, #13189, .F. ) ;
#23688=EDGE_CURVE ( 'NONE', #2128, #39376, #30380, .T. ) ;
#23733=ORIENTED_EDGE ( 'NONE', *, *, #24219, .F. ) ;
#23736=B_SPLINE_CURVE_WITH_KNOTS ( 'NONE', 3,
 ( #18333, #35413, #4189, #14686, #14914, #15364, #29268, #43183, #44319, #44089, #2109, #1884, #26755, #5754, #40437, #15811, #9416, #33335, #12854, #5535, #30172, #12399, #29945, #37214, #12630, #16037, #23107, #23328, #36316, #43858, #5086, #26528 ),
 .UNSPECIFIED., .F., .F.,
 ( 4, 2, 2, 2, 1, 1, 1, 1, 2, 2, 2, 2, 1, 1, 1, 1, 2, 2, 2, 4 ),
 ( 0.000000000000000000, 0.1249999999996142253, 0.1874999999994223787, 0.2187499999993277600, 0.2343749999992789101, 0.2421874999992546795, 0.2460937499992454647, 0.2480468749992408850, 0.2490234374992384980, 0.2499999999992360555, 0.3749999999992827404, 0.4374999999993081645, 0.4687499999993228195, 0.4843749999993324229, 0.4921874999993394173, 0.4960937499993454125, 0.4980468749993482436, 0.4999999999993510746, 0.7499999999996754818, 1.000000000000000000 ),
 .UNSPECIFIED. ) ;
#23748=CARTESIAN_POINT ( 'NONE',  ( 61.63318325272354770, -19.46990085680238636, -10.89321520033831447 ) ) ;
#23752=VERTEX_POINT ( 'NONE', #1083 ) ;
#23759=CARTESIAN_POINT ( 'NONE',  ( 62.93574133341893173, -12.59213563260223800, -10.20028763956079132 ) ) ;
#23792=CARTESIAN_POINT ( 'NONE',  ( 59.75121349346655109, -13.58877957849837870, -19.38162691376808411 ) ) ;
#23832=DIRECTION ( 'NONE',  ( 0.000000000000000000, 0.000000000000000000, -1.000000000000000000 ) ) ;
#23835=ORIENTED_EDGE ( 'NONE', *, *, #469, .F. ) ;
#23840=CARTESIAN_POINT ( 'NONE',  ( -1.307700928565892706, -16.07486664983353819, -18.19321520033831519 ) ) ;
#23858=DIRECTION ( 'NONE',  ( 0.000000000000000000, 0.000000000000000000, -1.000000000000000000 ) ) ;
#23878=EDGE_LOOP ( 'NONE', ( #9542, #38560, #30739, #7087 ) ) ;
#23894=VERTEX_POINT ( 'NONE', #11805 ) ;
#23911=DIRECTION ( 'NONE',  ( 0.000000000000000000, 0.000000000000000000, 1.000000000000000000 ) ) ;
#23912=DIRECTION ( 'NONE',  ( -0.9498278979187092519, -0.3127730236694430399, 0.000000000000000000 ) ) ;
#23935=DIRECTION ( 'NONE',  ( -0.9908103287288504424, 0.1352586133457950590, 0.000000000000000000 ) ) ;
#23951=ORIENTED_EDGE ( 'NONE', *, *, #43477, .T. ) ;
#23979=EDGE_LOOP ( 'NONE', ( #25577, #13532, #7264, #20963 ) ) ;
#23991=LINE ( 'NONE', #37427, #30238 ) ;
#23993=CARTESIAN_POINT ( 'NONE',  ( 59.62174278132244609, -14.86814543204979344, -18.19321520033831519 ) ) ;
#24001=FACE_OUTER_BOUND ( 'NONE', #14034, .T. ) ;
#24014=CARTESIAN_POINT ( 'NONE',  ( 59.62174278132245320, -14.86814543204979344, -19.39321520033831803 ) ) ;
#24036=VECTOR ( 'NONE', #42720, 1000.000000000000000 ) ;
#24045=CARTESIAN_POINT ( 'NONE',  ( 60.06931813437628875, -14.72076136720887085, -8.603412892520118760 ) ) ;
#24046=CARTESIAN_POINT ( 'NONE',  ( 62.79048817247115721, -3.396818809258673966, -7.619046670169436375 ) ) ;
#24055=DIRECTION ( 'NONE',  ( -0.4225728684367167642, 0.9063289528979890930, 0.000000000000000000 ) ) ;
#24108=AXIS2_PLACEMENT_3D ( 'NONE', #28603, #11273, #25181 ) ;
#24109=CYLINDRICAL_SURFACE ( 'NONE', #4832, 11.00000000000000000 ) ;
#24112=ORIENTED_EDGE ( 'NONE', *, *, #38229, .T. ) ;
#24122=CIRCLE ( 'NONE', #20477, 8.800000000000000711 ) ;
#24134=VERTEX_POINT ( 'NONE', #2652 ) ;
#24149=LINE ( 'NONE', #41700, #3812 ) ;
#24167=VERTEX_POINT ( 'NONE', #33882 ) ;
#24175=ORIENTED_EDGE ( 'NONE', *, *, #34484, .T. ) ;
#24192=VERTEX_POINT ( 'NONE', #23652 ) ;
#24206=AXIS2_PLACEMENT_3D ( 'NONE', #10980, #38777, #4348 ) ;
#24209=DIRECTION ( 'NONE',  ( -0.7962509850245453880, -0.6049664196031389052, 0.000000000000000000 ) ) ;
#24219=EDGE_CURVE ( 'NONE', #10084, #18111, #43715, .T. ) ;
#24239=ORIENTED_EDGE ( 'NONE', *, *, #17797, .T. ) ;
#24258=ORIENTED_EDGE ( 'NONE', *, *, #32827, .T. ) ;
#24259=CARTESIAN_POINT ( 'NONE',  ( 61.63318325272354770, -19.46990085680238636, -12.39321520033831447 ) ) ;
#24268=CARTESIAN_POINT ( 'NONE',  ( 59.24641515291911986, -13.72835195454734425, -7.393215200338313586 ) ) ;
#24269=CARTESIAN_POINT ( 'NONE',  ( 63.36814607564562607, -3.176177366285224846, -7.750926265059984388 ) ) ;
#24276=EDGE_LOOP ( 'NONE', ( #14348, #27928, #11580, #40827 ) ) ;
#24306=EDGE_LOOP ( 'NONE', ( #9999, #11625, #18273, #8436 ) ) ;
#24326=CARTESIAN_POINT ( 'NONE',  ( 62.88020800785245967, -12.58185084616640204, -16.61333427033593679 ) ) ;
#24333=CARTESIAN_POINT ( 'NONE',  ( 46.47434218039879283, -17.93412427487546523, -19.39321520033831447 ) ) ;
#24370=CARTESIAN_POINT ( 'NONE',  ( -13.55927693411048196, -4.790939057849996630, -8.800639967176238088 ) ) ;
#24378=AXIS2_PLACEMENT_3D ( 'NONE', #19279, #44586, #40482 ) ;
#24401=DIRECTION ( 'NONE',  ( -0.9908103287288504424, 0.1352586133457950313, 0.000000000000000000 ) ) ;
#24415=CARTESIAN_POINT ( 'NONE',  ( 62.63983398123977508, -12.53686781608317524, -10.05482766178462306 ) ) ;
#24424=DIRECTION ( 'NONE',  ( 0.000000000000000000, 0.000000000000000000, 1.000000000000000000 ) ) ;
#24432=( BOUNDED_SURFACE ( )  B_SPLINE_SURFACE ( 3, 2, ( 
 ( #11184, #31912, #43085 ),
 ( #677, #32137, #905 ),
 ( #14825, #28736, #42640 ),
 ( #32797, #11409, #42864 ),
 ( #7975, #21883, #4547 ),
 ( #18474, #15047, #11624 ) ),
 .UNSPECIFIED., .F., .F., .F. ) 
 B_SPLINE_SURFACE_WITH_KNOTS ( ( 4, 2, 4 ),
 ( 3, 3 ),
 ( 4.712388980384689674, 5.119002572906850013, 5.525616165429000581 ),
 ( 0.000000000000000000, 1.000000000000000000 ),
 .UNSPECIFIED. ) 
 GEOMETRIC_REPRESENTATION_ITEM ( )  RATIONAL_B_SPLINE_SURFACE ( (
 ( 1.000000000000000000, 0.7071067811865480168, 1.000000000000000000),
 ( 1.000000000000000000, 0.6811935452788959733, 1.000000000000000000),
 ( 1.000000000000000000, 0.6537392461962540091, 1.000000000000000000),
 ( 1.000000000000000000, 0.5999941409395589398, 1.000000000000000000),
 ( 1.000000000000000000, 0.5737032816804560342, 1.000000000000000000),
 ( 1.000000000000000000, 0.5507978985089549973, 1.000000000000000000) ) ) 
 REPRESENTATION_ITEM ( '' )  SURFACE ( )  );
#24449=DIRECTION ( 'NONE',  ( -0.9908103287288505534, 0.1352586133457951978, 0.000000000000000000 ) ) ;
#24454=DIRECTION ( 'NONE',  ( 0.4225728684367169308, -0.9063289528979889820, 0.000000000000000000 ) ) ;
#24469=CARTESIAN_POINT ( 'NONE',  ( 69.69189222815028018, -41.76310523276638520, -19.39321520033831447 ) ) ;
#24478=CARTESIAN_POINT ( 'NONE',  ( 75.63675420052337017, -42.57465691284114939, -19.39321520033831447 ) ) ;
#24484=AXIS2_PLACEMENT_3D ( 'NONE', #29025, #26275, #22623 ) ;
#24528=ORIENTED_EDGE ( 'NONE', *, *, #2187, .F. ) ;
#24534=CARTESIAN_POINT ( 'NONE',  ( 67.93084693336861335, 0.8442783687841282081, -9.853887653298288640 ) ) ;
#24541=CARTESIAN_POINT ( 'NONE',  ( 60.94960279574944195, -12.50265280191595529, -17.24776159451941382 ) ) ;
#24547=DIRECTION ( 'NONE',  ( 0.9908103287288504424, -0.1352586133457950590, 0.000000000000000000 ) ) ;
#24566=TOROIDAL_SURFACE ( 'NONE', #3435, 4.500000000000000000, 0.5000000000000000000 ) ;
#24584=VERTEX_POINT ( 'NONE', #17370 ) ;
#24586=ADVANCED_FACE ( 'NONE', ( #31259 ), #10091, .T. ) ;
#24587=CARTESIAN_POINT ( 'NONE',  ( 81.52050388106540879, 0.5255923868638483487, -16.39321520033831447 ) ) ;
#24609=DIRECTION ( 'NONE',  ( 0.9908103287288504424, -0.1352586133457950313, 0.000000000000000000 ) ) ;
#24617=CARTESIAN_POINT ( 'NONE',  ( 66.21635238248168775, -14.64006919827764364, -16.51222081763639338 ) ) ;
#24629=DIRECTION ( 'NONE',  ( -0.9908103287288511085, 0.1352586133457904793, 0.000000000000000000 ) ) ;
#24630=CARTESIAN_POINT ( 'NONE',  ( 61.63318325272354770, -19.46990085680238636, -15.89321520033831447 ) ) ;
#24633=ORIENTED_EDGE ( 'NONE', *, *, #2994, .F. ) ;
#24669=CARTESIAN_POINT ( 'NONE',  ( 60.99435512697147033, -13.32931833351155326, -19.27180043387577157 ) ) ;
#24705=ORIENTED_EDGE ( 'NONE', *, *, #42046, .T. ) ;
#24721=CARTESIAN_POINT ( 'NONE',  ( 64.46696884417693241, -15.35047623415474405, -15.89321305673442986 ) ) ;
#24757=CARTESIAN_POINT ( 'NONE',  ( 63.74703025577719018, -40.95155355269160680, -15.89321520033831447 ) ) ;
#24778=CARTESIAN_POINT ( 'NONE',  ( 67.08264006073221708, -20.21382323020432992, -10.39321520033831625 ) ) ;
#24826=ORIENTED_EDGE ( 'NONE', *, *, #19286, .T. ) ;
#24837=CARTESIAN_POINT ( 'NONE',  ( 65.71132926441107713, -16.34206498534276264, -16.79547554155828593 ) ) ;
#24851=DIRECTION ( 'NONE',  ( 0.000000000000000000, 0.000000000000000000, 1.000000000000000000 ) ) ;
#24872=CARTESIAN_POINT ( 'NONE',  ( 55.68041887817022939, -39.85035523279287162, -7.393215200338315363 ) ) ;
#24873=AXIS2_PLACEMENT_3D ( 'NONE', #31226, #37845, #37628 ) ;
#24911=EDGE_CURVE ( 'NONE', #5770, #30504, #44970, .T. ) ;
#24914=ORIENTED_EDGE ( 'NONE', *, *, #43534, .F. ) ;
#24926=DIRECTION ( 'NONE',  ( 0.000000000000000000, 0.000000000000000000, -1.000000000000000000 ) ) ;
#24956=CARTESIAN_POINT ( 'NONE',  ( 64.43454729525839753, -13.05486520922822713, -11.18801556346294390 ) ) ;
#24976=CARTESIAN_POINT ( 'NONE',  ( -7.917624645353497748, -12.21642755857638818, -8.593215200338315540 ) ) ;
#24984=CARTESIAN_POINT ( 'NONE',  ( 66.50565249108366572, -35.53029877516337365, -12.39321520033831447 ) ) ;
#24987=DIRECTION ( 'NONE',  ( 0.7962509850245451659, 0.6049664196031394603, 0.000000000000000000 ) ) ;
#24988=CARTESIAN_POINT ( 'NONE',  ( 60.06931813437629586, -14.72076136720887085, -18.18301750815651374 ) ) ;
#24989=DIRECTION ( 'NONE',  ( 0.9908103287288504424, -0.1352586133457950035, 0.000000000000000000 ) ) ;
#25009=EDGE_CURVE ( 'NONE', #29964, #18680, #42277, .T. ) ;
#25017=VECTOR ( 'NONE', #29120, 1000.000000000000000 ) ;
#25037=DIRECTION ( 'NONE',  ( 0.9908103287288504424, -0.1352586133457950590, 0.000000000000000000 ) ) ;
#25066=CARTESIAN_POINT ( 'NONE',  ( 59.75121349346655109, -13.58877957849837692, -19.38162691376808411 ) ) ;
#25067=CARTESIAN_POINT ( 'NONE',  ( 65.01222975847794316, -15.66120467700027064, -17.43105922203487523 ) ) ;
#25071=ORIENTED_EDGE ( 'NONE', *, *, #8947, .T. ) ;
#25101=EDGE_CURVE ( 'NONE', #2056, #17567, #29868, .T. ) ;
#25117=EDGE_CURVE ( 'NONE', #14190, #5770, #11638, .T. ) ;
#25124=EDGE_CURVE ( 'NONE', #36955, #37929, #32034, .T. ) ;
#25127=CARTESIAN_POINT ( 'NONE',  ( -13.78505786849281911, -3.796669023460694792, -17.89321520033831447 ) ) ;
#25146=ORIENTED_EDGE ( 'NONE', *, *, #34063, .T. ) ;
#25159=DIRECTION ( 'NONE',  ( 0.000000000000000000, 0.000000000000000000, -1.000000000000000000 ) ) ;
#25160=DIRECTION ( 'NONE',  ( -0.9908103287288504424, 0.1352586133457950590, 0.000000000000000000 ) ) ;
#25181=DIRECTION ( 'NONE',  ( -0.9908103287288504424, 0.1352586133457958917, 0.000000000000000000 ) ) ;
#25186=CARTESIAN_POINT ( 'NONE',  ( 65.46440686121715657, -13.61036171439920928, -12.26818186452783266 ) ) ;
#25208=CARTESIAN_POINT ( 'NONE',  ( 61.63318325272354770, -19.46990085680238636, -19.39321520033831447 ) ) ;
#25220=CARTESIAN_POINT ( 'NONE',  ( 64.85972373664627355, -13.90976778618263410, -9.092962798488864351 ) ) ;
#25266=CARTESIAN_POINT ( 'NONE',  ( 66.31675885524160208, -2.050240359669329937, -8.986641377623520555 ) ) ;
#25290=CARTESIAN_POINT ( 'NONE',  ( 59.58306117764126952, -13.63527223977064295, -7.397078708827238280 ) ) ;
#25295=CARTESIAN_POINT ( 'NONE',  ( 61.00841592940014380, -13.32659487457196335, -19.27059286807817884 ) ) ;
#25296=VECTOR ( 'NONE', #9978, 999.9999999999998863 ) ;
#25309=CARTESIAN_POINT ( 'NONE',  ( 63.56235174433628998, -1.192518024930046661, -9.408727405721505122 ) ) ;
#25317=EDGE_CURVE ( 'NONE', #31011, #14190, #36686, .T. ) ;
#25331=CARTESIAN_POINT ( 'NONE',  ( 69.69189222815028018, -41.76310523276638520, -12.39321520033831447 ) ) ;
#25332=DIRECTION ( 'NONE',  ( 0.000000000000000000, 0.000000000000000000, -1.000000000000000000 ) ) ;
#25349=CARTESIAN_POINT ( 'NONE',  ( -6.962123463324020101, -11.49046785505261248, -18.19321520033831519 ) ) ;
#25362=DIRECTION ( 'NONE',  ( 0.000000000000000000, 0.000000000000000000, -1.000000000000000000 ) ) ;
#25373=EDGE_CURVE ( 'NONE', #30249, #41341, #40355, .T. ) ;
#25377=ORIENTED_EDGE ( 'NONE', *, *, #44678, .T. ) ;
#25407=FACE_OUTER_BOUND ( 'NONE', #19568, .T. ) ;
#25412=DIRECTION ( 'NONE',  ( 0.000000000000000000, 0.000000000000000000, -1.000000000000000000 ) ) ;
#25421=ORIENTED_EDGE ( 'NONE', *, *, #490, .T. ) ;
#25437=VECTOR ( 'NONE', #14083, 1000.000000000000000 ) ;
#25439=CARTESIAN_POINT ( 'NONE',  ( -1.637506834317598026, -6.775152287193681566, -19.39321520033831447 ) ) ;
#25445=CARTESIAN_POINT ( 'NONE',  ( 27.78057335388972504, -13.48551096636548330, -19.39321520033831447 ) ) ;
#25447=CARTESIAN_POINT ( 'NONE',  ( 61.87551538731119649, -14.47097590406426093, -8.981403309440874949 ) ) ;
#25463=CARTESIAN_POINT ( 'NONE',  ( -13.56828337869067269, -4.779084862086131480, -8.846323889245468308 ) ) ;
#25491=CARTESIAN_POINT ( 'NONE',  ( -13.52882246642779940, -4.831022935409089669, -8.722530528169237130 ) ) ;
#25494=CARTESIAN_POINT ( 'NONE',  ( 66.02316373260774185, -0.1478461060746093236, -16.39321520033831447 ) ) ;
#25516=AXIS2_PLACEMENT_3D ( 'NONE', #4107, #472, #15061 ) ;
#25519=CARTESIAN_POINT ( 'NONE',  ( 64.39944321480182055, -15.22860971205249569, -17.87854327940120669 ) ) ;
#25534=VECTOR ( 'NONE', #41833, 1000.000000000000000 ) ;
#25550=DIRECTION ( 'NONE',  ( 0.1352586133457950590, 0.9908103287288504424, 0.000000000000000000 ) ) ;
#25577=ORIENTED_EDGE ( 'NONE', *, *, #2440, .T. ) ;
#25579=AXIS2_PLACEMENT_3D ( 'NONE', #18794, #15373, #22880 ) ;
#25608=EDGE_CURVE ( 'NONE', #17168, #16401, #18996, .T. ) ;
#25618=PLANE ( 'NONE',  #23353 ) ;
#25624=ADVANCED_FACE ( 'NONE', ( #9996 ), #5701, .T. ) ;
#25630=EDGE_CURVE ( 'NONE', #20781, #36610, #23366, .T. ) ;
#25656=AXIS2_PLACEMENT_3D ( 'NONE', #36501, #44042, #44275 ) ;
#25659=AXIS2_PLACEMENT_3D ( 'NONE', #40650, #19898, #5742 ) ;
#25663=CARTESIAN_POINT ( 'NONE',  ( 64.96812053257905006, -13.31534605384092984, -15.09338587514541352 ) ) ;
#25665=CARTESIAN_POINT ( 'NONE',  ( -13.23804852390367337, -4.035795733041972255, -7.689295463341079717 ) ) ;
#25668=AXIS2_PLACEMENT_3D ( 'NONE', #29142, #22303, #31654 ) ;
#25669=CARTESIAN_POINT ( 'NONE',  ( -1.637506834317628890, -6.775152287193632716, -18.06807615187975102 ) ) ;
#25670=CARTESIAN_POINT ( 'NONE',  ( 62.99198783763660003, -14.62836571490823978, -8.152764136444947241 ) ) ;
#25695=FACE_OUTER_BOUND ( 'NONE', #42110, .T. ) ;
#25705=VECTOR ( 'NONE', #18536, 1000.000000000000000 ) ;
#25714=CARTESIAN_POINT ( 'NONE',  ( -13.50772587709714578, -4.858790063452675057, -8.690212664598012893 ) ) ;
#25756=STYLED_ITEM('',(#45162),#21433);
#25780=CARTESIAN_POINT ( 'NONE',  ( 64.71874404463645192, -15.46959023120085064, -16.14765141715094998 ) ) ;
#25838=VERTEX_POINT ( 'NONE', #5474 ) ;
#25849=CARTESIAN_POINT ( 'NONE',  ( -1.637506834317598026, -6.775152287193681566, -8.893215200338314474 ) ) ;
#25865=AXIS2_PLACEMENT_3D ( 'NONE', #2388, #33846, #22468 ) ;
#25884=CARTESIAN_POINT ( 'NONE',  ( 65.18805517862392662, -13.43643968393412358, -14.85905743718944727 ) ) ;
#25889=CARTESIAN_POINT ( 'NONE',  ( -2.026929177228822709, -6.892617277590884051, -18.91977777107071645 ) ) ;
#25890=CARTESIAN_POINT ( 'NONE',  ( 65.38099912316067730, -15.98743937505324553, -9.669194438446968576 ) ) ;
#25910=CARTESIAN_POINT ( 'NONE',  ( -13.61777589163126123, -4.713943292400020191, -18.99709152357623410 ) ) ;
#25923=PRODUCT_CONTEXT ( 'NONE', #16044, 'mechanical' ) ;
#25936=CARTESIAN_POINT ( 'NONE',  ( 65.10175888621736817, -2.513761081768071559, -8.357200856923110877 ) ) ;
#25975=FILL_AREA_STYLE ('',( #1343 ) ) ;
#25977=MECHANICAL_DESIGN_GEOMETRIC_PRESENTATION_REPRESENTATION('',(#2631),#17104);
#25986=ORIENTED_EDGE ( 'NONE', *, *, #18903, .F. ) ;
#25991=ORIENTED_EDGE ( 'NONE', *, *, #37255, .F. ) ;
#25993=EDGE_CURVE ( 'NONE', #8541, #23633, #10441, .T. ) ;
#25999=VECTOR ( 'NONE', #44599, 1000.000000000000000 ) ;
#26033=EDGE_LOOP ( 'NONE', ( #9181, #30912, #12967, #38155, #38089 ) ) ;
#26038=CARTESIAN_POINT ( 'NONE',  ( 64.58074566301215214, -15.42874415904032936, -10.76541893930477123 ) ) ;
#26048=CARTESIAN_POINT ( 'NONE',  ( 66.27237322303049893, -14.92696213753554524, -16.39321520033831447 ) ) ;
#26075=LINE ( 'NONE', #15816, #15737 ) ;
#26081=CARTESIAN_POINT ( 'NONE',  ( 72.84358186299090221, -48.24900165852266554, -12.39321520033831447 ) ) ;
#26101=FACE_OUTER_BOUND ( 'NONE', #5133, .T. ) ;
#26104=CARTESIAN_POINT ( 'NONE',  ( 65.00799056132680676, -13.33714338733787663, -15.05121535635604779 ) ) ;
#26111=CARTESIAN_POINT ( 'NONE',  ( 65.75155193749419880, -0.2203213019380833582, -10.39321520033831270 ) ) ;
#26112=CARTESIAN_POINT ( 'NONE',  ( -1.971352495715082309, -6.875908495535235865, -18.85450084843566643 ) ) ;
#26118=CARTESIAN_POINT ( 'NONE',  ( 69.69189222815028018, -41.76310523276638520, -15.89321520033831447 ) ) ;
#26126=DIRECTION ( 'NONE',  ( -0.6049664196031393493, 0.7962509850245451659, 0.000000000000000000 ) ) ;
#26139=CARTESIAN_POINT ( 'NONE',  ( 74.82520252044861309, -48.51951888521425360, -12.39321520033831447 ) ) ;
#26160=CARTESIAN_POINT ( 'NONE',  ( 68.14371629974728251, -1.351251493923715685, -16.39321520033831447 ) ) ;
#26166=LINE ( 'NONE', #32545, #35452 ) ;
#26194=VERTEX_POINT ( 'NONE', #42406 ) ;
#26239=CARTESIAN_POINT ( 'NONE',  ( 60.53937939559665438, -4.256997083809236138, 68.32805411424035924 ) ) ;
#26246=CARTESIAN_POINT ( 'NONE',  ( 42.36021970110777346, -12.73296999994090584, -8.893215200338314474 ) ) ;
#26258=AXIS2_PLACEMENT_3D ( 'NONE', #2856, #23858, #30229 ) ;
#26275=DIRECTION ( 'NONE',  ( 0.000000000000000000, 0.000000000000000000, -1.000000000000000000 ) ) ;
#26278=AXIS2_PLACEMENT_3D ( 'NONE', #32109, #21184, #41943 ) ;
#26309=DIRECTION ( 'NONE',  ( -1.000000000000000000, 0.000000000000000000, 0.000000000000000000 ) ) ;
#26316=CIRCLE ( 'NONE', #37965, 1.499999999999998002 ) ;
#26341=CARTESIAN_POINT ( 'NONE',  ( 65.97129655291890060, -0.1603451389117774017, -10.39321520033831270 ) ) ;
#26344=DIRECTION ( 'NONE',  ( -0.9908103287288505534, 0.1352586133457950868, 0.000000000000000000 ) ) ;
#26347=VERTEX_POINT ( 'NONE', #18682 ) ;
#26349=CARTESIAN_POINT ( 'NONE',  ( 66.30460113213176498, -14.82332738410570805, -10.39321520033831092 ) ) ;
#26360=CARTESIAN_POINT ( 'NONE',  ( -13.32377113153209791, -5.100909530930219482, -19.39321520033831803 ) ) ;
#26385=CARTESIAN_POINT ( 'NONE',  ( 62.95628177081277954, -3.333487351105247409, -7.653476909290080066 ) ) ;
#26387=CARTESIAN_POINT ( 'NONE',  ( 67.88234748603528601, -0.4879875857827546959, -16.39321520033831447 ) ) ;
#26406=DIRECTION ( 'NONE',  ( -0.9908103287288497762, 0.1352586133458010265, 0.000000000000000000 ) ) ;
#26428=EDGE_CURVE ( 'NONE', #11018, #854, #12297, .T. ) ;
#26449=EDGE_CURVE ( 'NONE', #25838, #40192, #21929, .T. ) ;
#26452=CARTESIAN_POINT ( 'NONE',  ( 60.34146317132753978, -13.36775875599912844, -7.393215200338315363 ) ) ;
#26478=PLANE ( 'NONE',  #18435 ) ;
#26503=EDGE_CURVE ( 'NONE', #43140, #11788, #5906, .T. ) ;
#26511=EDGE_CURVE ( 'NONE', #14190, #11722, #7244, .T. ) ;
#26516=CYLINDRICAL_SURFACE ( 'NONE', #32904, 1.199999999999999512 ) ;
#26528=CARTESIAN_POINT ( 'NONE',  ( 68.14371629974728251, -1.351251493923715685, -16.39321520033831447 ) ) ;
#26567=CARTESIAN_POINT ( 'NONE',  ( 67.74656486299329572, -0.3633886386785405986, -10.39321520033831625 ) ) ;
#26574=DIRECTION ( 'NONE',  ( -0.9908103287288505534, 0.1352586133457945317, 0.000000000000000000 ) ) ;
#26581=FACE_OUTER_BOUND ( 'NONE', #34417, .T. ) ;
#26583=ADVANCED_FACE ( 'NONE', ( #30682 ), #10167, .T. ) ;
#26585=CARTESIAN_POINT ( 'NONE',  ( -13.56828339430762398, -4.779084841531242134, -17.94044720194083808 ) ) ;
#26628=CIRCLE ( 'NONE', #6977, 1.199999999999999734 ) ;
#26666=CARTESIAN_POINT ( 'NONE',  ( 74.47157298427187300, -3.053873105668316601, -7.147228641687434880 ) ) ;
#26685=EDGE_CURVE ( 'NONE', #38550, #6765, #41850, .T. ) ;
#26699=DIRECTION ( 'NONE',  ( 0.9908103287288505534, -0.1352586133457944206, 0.000000000000000000 ) ) ;
#26727=AXIS2_PLACEMENT_3D ( 'NONE', #14727, #31820, #24987 ) ;
#26736=CYLINDRICAL_SURFACE ( 'NONE', #4329, 25.00000000000000355 ) ;
#26738=ORIENTED_EDGE ( 'NONE', *, *, #401, .T. ) ;
#26741=EDGE_CURVE ( 'NONE', #16290, #22059, #10293, .T. ) ;
#26743=DIRECTION ( 'NONE',  ( 0.9908103287288504424, -0.1352586133457958917, 0.000000000000000000 ) ) ;
#26747=AXIS2_PLACEMENT_3D ( 'NONE', #21734, #531, #25160 ) ;
#26749=VERTEX_POINT ( 'NONE', #1006 ) ;
#26752=CARTESIAN_POINT ( 'NONE',  ( 59.95220766929347889, -14.75932518950460981, -19.37269899291708697 ) ) ;
#26755=CARTESIAN_POINT ( 'NONE',  ( 62.61495183759026162, -3.463885907106070139, -19.20140212329127039 ) ) ;
#26760=CARTESIAN_POINT ( 'NONE',  ( -2.793826376213096818, -7.122619984182616548, -7.420824263456360370 ) ) ;
#26777=EDGE_CURVE ( 'NONE', #39048, #31742, #37549, .T. ) ;
#26784=DIRECTION ( 'NONE',  ( 0.1352586133458071049, 0.9908103287288489991, 0.000000000000000000 ) ) ;
#26800=FACE_BOUND ( 'NONE', #38804, .T. ) ;
#26808=CARTESIAN_POINT ( 'NONE',  ( 9.052690036452151645, -4.182915634381243919, -19.39321520033831447 ) ) ;
#26819=EDGE_LOOP ( 'NONE', ( #16826, #40170, #26922, #11669, #716, #28787, #37553, #23951, #7088, #28905 ) ) ;
#26823=ADVANCED_FACE ( 'NONE', ( #13493 ), #34655, .F. ) ;
#26834=ORIENTED_EDGE ( 'NONE', *, *, #14554, .T. ) ;
#26922=ORIENTED_EDGE ( 'NONE', *, *, #44897, .T. ) ;
#26931=EDGE_LOOP ( 'NONE', ( #4834, #28086, #21295, #25986 ) ) ;
#26990=ORIENTED_EDGE ( 'NONE', *, *, #14827, .T. ) ;
#27010=TOROIDAL_SURFACE ( 'NONE', #26258, 26.50000000000000000, 1.500000000000000000 ) ;
#27011=CARTESIAN_POINT ( 'NONE',  ( 64.24243542014160369, -41.01918285936451269, -10.89321520033831447 ) ) ;
#27012=VECTOR ( 'NONE', #36470, 1000.000000000000000 ) ;
#27023=DIRECTION ( 'NONE',  ( -0.9908103287288505534, 0.1352586133457945317, 0.000000000000000000 ) ) ;
#27028=ORIENTED_EDGE ( 'NONE', *, *, #9456, .F. ) ;
#27104=AXIS2_PLACEMENT_3D ( 'NONE', #17352, #35088, #34861 ) ;
#27124=AXIS2_PLACEMENT_3D ( 'NONE', #38340, #24449, #38128 ) ;
#27160=FACE_OUTER_BOUND ( 'NONE', #16720, .T. ) ;
#27164=CIRCLE ( 'NONE', #14041, 1.500000000000000666 ) ;
#27166=AXIS2_PLACEMENT_3D ( 'NONE', #44368, #34083, #2850 ) ;
#27171=CARTESIAN_POINT ( 'NONE',  ( 60.02417077683579549, -12.62998352332487606, -9.398546866638605835 ) ) ;
#27176=AXIS2_PLACEMENT_3D ( 'NONE', #43650, #26784, #9445 ) ;
#27184=EDGE_CURVE ( 'NONE', #42225, #11850, #29117, .T. ) ;
#27202=VERTEX_POINT ( 'NONE', #32146 ) ;
#27205=CARTESIAN_POINT ( 'NONE',  ( 66.58723489636778936, -20.14619392353143112, -10.89321520033831447 ) ) ;
#27208=CARTESIAN_POINT ( 'NONE',  ( 74.64594387179452895, -42.43939829949535181, -10.39321520033831625 ) ) ;
#27214=CARTESIAN_POINT ( 'NONE',  ( 42.36021970110777346, -12.73296999994090584, -8.893215200338314474 ) ) ;
#27231=VECTOR ( 'NONE', #31670, 1000.000000000000114 ) ;
#27240=CARTESIAN_POINT ( 'NONE',  ( 60.53937939559665438, -4.256997083809236138, -7.393215200338315363 ) ) ;
#27247=EDGE_LOOP ( 'NONE', ( #10977, #1153, #43977, #13953, #40900, #17178, #24258, #16850, #23122, #36330 ) ) ;
#27283=ORIENTED_EDGE ( 'NONE', *, *, #38229, .F. ) ;
#27308=DIRECTION ( 'NONE',  ( 0.9908103287288505534, -0.1352586133457944206, 0.000000000000000000 ) ) ;
#27348=AXIS2_PLACEMENT_3D ( 'NONE', #28021, #38260, #14778 ) ;
#27381=DIRECTION ( 'NONE',  ( 0.000000000000000000, 0.000000000000000000, 1.000000000000000000 ) ) ;
#27418=CARTESIAN_POINT ( 'NONE',  ( 31.16203868753470019, 11.28474725185576055, -19.39321520033831447 ) ) ;
#27420=VERTEX_POINT ( 'NONE', #12090 ) ;
#27432=FACE_OUTER_BOUND ( 'NONE', #750, .T. ) ;
#27454=ORIENTED_EDGE ( 'NONE', *, *, #18643, .T. ) ;
#27464=DIRECTION ( 'NONE',  ( -0.9908103287288499983, 0.1352586133457985007, -3.469446951953614978E-15 ) ) ;
#27474=CARTESIAN_POINT ( 'NONE',  ( 63.43088374006683239, -46.96404483173760269, -10.39321520033831625 ) ) ;
#27476=CARTESIAN_POINT ( 'NONE',  ( 71.62928943233082180, 0.3619606153155430217, -14.39321520033831625 ) ) ;
#27477=CARTESIAN_POINT ( 'NONE',  ( -2.511237114481913668, -7.038084878006822365, -19.27282189517453048 ) ) ;
#27481=ORIENTED_EDGE ( 'NONE', *, *, #18422, .T. ) ;
#27493=DIRECTION ( 'NONE',  ( -0.9908103287288504424, 0.1352586133457954476, 0.000000000000000000 ) ) ;
#27501=VERTEX_POINT ( 'NONE', #32810 ) ;
#27548=CARTESIAN_POINT ( 'NONE',  ( 69.69189222815028018, -41.76310523276638520, -7.393215200338315363 ) ) ;
#27575=CARTESIAN_POINT ( 'NONE',  ( -13.56828337869107948, -4.779084862085587915, -8.893215200338321580 ) ) ;
#27613=DIRECTION ( 'NONE',  ( 0.000000000000000000, 0.000000000000000000, 1.000000000000000000 ) ) ;
#27620=ORIENTED_EDGE ( 'NONE', *, *, #4845, .F. ) ;
#27637=DIRECTION ( 'NONE',  ( 0.000000000000000000, 0.000000000000000000, -1.000000000000000000 ) ) ;
#27659=CARTESIAN_POINT ( 'NONE',  ( 31.16856251326852956, -20.50830283073288385, -19.39321520033831447 ) ) ;
#27730=( BOUNDED_CURVE ( )  B_SPLINE_CURVE ( 3, ( #11401, #11619, #25309, #15041 ),
 .UNSPECIFIED., .F., .T. ) 
 B_SPLINE_CURVE_WITH_KNOTS ( ( 4, 4 ),
 ( 1.570796326794895004, 2.173987732404564888 ),
 .UNSPECIFIED. ) 
 CURVE ( )  GEOMETRIC_REPRESENTATION_ITEM ( )  RATIONAL_B_SPLINE_CURVE ( ( 1.000000000000000000, 0.9699091404214869039, 0.9699091404214869039, 1.000000000000000000 ) ) 
 REPRESENTATION_ITEM ( '' )  );
#27744=DIRECTION ( 'NONE',  ( -0.9908103287288504424, 0.1352586133457951423, 0.000000000000000000 ) ) ;
#27746=CARTESIAN_POINT ( 'NONE',  ( 62.79269271256460172, -12.56645042133913392, -16.65519758901568181 ) ) ;
#27792=CARTESIAN_POINT ( 'NONE',  ( -13.78505786741674655, -3.796669018538534779, -8.660771829302781555 ) ) ;
#27797=CARTESIAN_POINT ( 'NONE',  ( 9.052690036452151645, -4.182915634381243919, -17.89321520033831447 ) ) ;
#27825=CIRCLE ( 'NONE', #17631, 1.500000000000001332 ) ;
#27870=CARTESIAN_POINT ( 'NONE',  ( -13.32377113153209791, -5.100909530930220370, -18.19321520033831874 ) ) ;
#27872=EDGE_LOOP ( 'NONE', ( #11039, #13428, #9816, #11158 ) ) ;
#27875=LINE ( 'NONE', #10770, #30715 ) ;
#27878=PLANE ( 'NONE',  #14101 ) ;
#27920=EDGE_LOOP ( 'NONE', ( #22595, #27620, #21714, #22502 ) ) ;
#27928=ORIENTED_EDGE ( 'NONE', *, *, #18431, .F. ) ;
#27935=CARTESIAN_POINT ( 'NONE',  ( 60.06931813437629586, -14.72076136720887085, -18.18301750815651374 ) ) ;
#27945=DIRECTION ( 'NONE',  ( 0.9908103287288528849, -0.1352586133457776008, 0.000000000000000000 ) ) ;
#27963=CARTESIAN_POINT ( 'NONE',  ( 68.27567836778572996, -1.300826558512744535, -10.52192843399248545 ) ) ;
#27981=ORIENTED_EDGE ( 'NONE', *, *, #38036, .F. ) ;
#28019=DIRECTION ( 'NONE',  ( 0.000000000000000000, 0.000000000000000000, -1.000000000000000000 ) ) ;
#28021=CARTESIAN_POINT ( 'NONE',  ( 71.99789814782840836, -24.87091310681484657, -18.19321520033831519 ) ) ;
#28030=CARTESIAN_POINT ( 'NONE',  ( 59.44377208703740223, -12.82110557137145967, -9.393546723914594665 ) ) ;
#28044=CARTESIAN_POINT ( 'NONE',  ( 64.20801161461099582, -15.17998946340411592, -16.19887345869426198 ) ) ;
#28056=CARTESIAN_POINT ( 'NONE',  ( 0.04488520489200759078, -6.166763362545027327, -8.593215200338315540 ) ) ;
#28069=EDGE_CURVE ( 'NONE', #19352, #22762, #44882, .T. ) ;
#28075=CARTESIAN_POINT ( 'NONE',  ( 59.77100663911058120, -14.81899367705580595, -18.19321520033832229 ) ) ;
#28076=ADVANCED_FACE ( 'NONE', ( #13194 ), #34363, .F. ) ;
#28086=ORIENTED_EDGE ( 'NONE', *, *, #17537, .F. ) ;
#28094=EDGE_LOOP ( 'NONE', ( #17961, #1079, #2183, #1405 ) ) ;
#28104=CIRCLE ( 'NONE', #2595, 1.500000000000001332 ) ;
#28108=ORIENTED_EDGE ( 'NONE', *, *, #16709, .T. ) ;
#28119=DIRECTION ( 'NONE',  ( -0.6049664196031393493, 0.7962509850245452769, 0.000000000000000000 ) ) ;
#28133=DIRECTION ( 'NONE',  ( -0.9908103287288504424, 0.1352586133457951423, 0.000000000000000000 ) ) ;
#28159=LINE ( 'NONE', #20201, #40484 ) ;
#28184=CARTESIAN_POINT ( 'NONE',  ( 63.12337091419462354, -3.603895683774054781, -9.393215200338314474 ) ) ;
#28193=FACE_OUTER_BOUND ( 'NONE', #20759, .T. ) ;
#28198=CARTESIAN_POINT ( 'NONE',  ( 61.63318325272354770, -19.46990085680238636, -19.39321520033831447 ) ) ;
#28215=LINE ( 'NONE', #35010, #37164 ) ;
#28224=UNCERTAINTY_MEASURE_WITH_UNIT (LENGTH_MEASURE( 1.000000000000000082E-05 ), #35773, 'distance_accuracy_value', 'NONE');
#28259=EDGE_CURVE ( 'NONE', #40326, #39449, #7442, .T. ) ;
#28266=CARTESIAN_POINT ( 'NONE',  ( 64.60369908702583075, -13.80855579193262805, -17.86746305170717619 ) ) ;
#28275=CIRCLE ( 'NONE', #43655, 1.199999999999999512 ) ;
#28279=DIRECTION ( 'NONE',  ( 0.000000000000000000, 0.000000000000000000, 1.000000000000000000 ) ) ;
#28280=DIRECTION ( 'NONE',  ( 0.000000000000000000, 0.000000000000000000, 1.000000000000000000 ) ) ;
#28295=CARTESIAN_POINT ( 'NONE',  ( 59.41811746136757222, -12.82955349636864639, -17.39310469171629947 ) ) ;
#28328=DIRECTION ( 'NONE',  ( 0.000000000000000000, 0.000000000000000000, 1.000000000000000000 ) ) ;
#28332=EDGE_LOOP ( 'NONE', ( #10490, #8158 ) ) ;
#28349=CARTESIAN_POINT ( 'NONE',  ( 61.63318325272354770, -19.46990085680238636, -10.89321520033831447 ) ) ;
#28378=CARTESIAN_POINT ( 'NONE',  ( 64.57113367631538381, -13.11585569015068664, -11.30697229492609068 ) ) ;
#28402=ADVANCED_FACE ( 'NONE', ( #36155 ), #21234, .T. ) ;
#28403=CARTESIAN_POINT ( 'NONE',  ( 62.74499803204670911, -14.59121584192012655, -9.399563555836040862 ) ) ;
#28440=( BOUNDED_CURVE ( )  B_SPLINE_CURVE ( 3, ( #37020, #16069, #5116, #12889 ),
 .UNSPECIFIED., .F., .F. ) 
 B_SPLINE_CURVE_WITH_KNOTS ( ( 4, 4 ),
 ( 4.712388980384689674, 5.608053774242550027 ),
 .UNSPECIFIED. ) 
 CURVE ( )  GEOMETRIC_REPRESENTATION_ITEM ( )  RATIONAL_B_SPLINE_CURVE ( ( 1.000000000000000000, 0.9342585459106650392, 0.9342585459106650392, 1.000000000000000000 ) ) 
 REPRESENTATION_ITEM ( '' )  );
#28445=AXIS2_PLACEMENT_3D ( 'NONE', #34963, #6966, #27945 ) ;
#28473=VECTOR ( 'NONE', #42748, 1000.000000000000114 ) ;
#28490=DIRECTION ( 'NONE',  ( 0.9908103287288504424, -0.1352586133457951423, 0.000000000000000000 ) ) ;
#28493=CARTESIAN_POINT ( 'NONE',  ( 61.96957081968723458, -13.30635274022726300, -19.04364310209689393 ) ) ;
#28521=ORIENTED_EDGE ( 'NONE', *, *, #16124, .F. ) ;
#28525=CARTESIAN_POINT ( 'NONE',  ( 64.73784058450603140, -41.08681216603740438, -16.39321520033831447 ) ) ;
#28568=DIRECTION ( 'NONE',  ( 0.000000000000000000, 0.000000000000000000, -1.000000000000000000 ) ) ;
#28573=VECTOR ( 'NONE', #42145, 1000.000000000000000 ) ;
#28602=CARTESIAN_POINT ( 'NONE',  ( 77.44400397045842510, -3.459648945705700473, -16.39321520033831447 ) ) ;
#28603=CARTESIAN_POINT ( 'NONE',  ( 67.08264006073221708, -20.21382323020432992, -15.89321520033831447 ) ) ;
#28640=CYLINDRICAL_SURFACE ( 'NONE', #34738, 0.4999999999999996669 ) ;
#28643=CARTESIAN_POINT ( 'NONE',  ( 62.52450766521648262, -14.54539169785276442, -9.275848827766759896 ) ) ;
#28669=ADVANCED_FACE ( 'NONE', ( #2399 ), #27010, .T. ) ;
#28688=ORIENTED_EDGE ( 'NONE', *, *, #38650, .F. ) ;
#28717=CARTESIAN_POINT ( 'NONE',  ( 66.40642813730079297, -14.77805237463982024, -16.29520547388278118 ) ) ;
#28730=FACE_OUTER_BOUND ( 'NONE', #556, .T. ) ;
#28736=CARTESIAN_POINT ( 'NONE',  ( 62.78977304965946615, -1.552730279056773410, -19.34404429361859457 ) ) ;
#28740=CARTESIAN_POINT ( 'NONE',  ( 60.06931813437629586, -14.72076136720887085, -8.603412892520118760 ) ) ;
#28766=ORIENTED_EDGE ( 'NONE', *, *, #10913, .T. ) ;
#28772=CARTESIAN_POINT ( 'NONE',  ( 60.37068618338318515, -13.41750073646542596, -19.35316885160253264 ) ) ;
#28787=ORIENTED_EDGE ( 'NONE', *, *, #26685, .F. ) ;
#28826=CARTESIAN_POINT ( 'NONE',  ( 60.91427317013496889, -14.50360402731953968, -18.09323085839352530 ) ) ;
#28853=CARTESIAN_POINT ( 'NONE',  ( -12.61278219666105649, -4.053125158562569830, -8.893215200338314474 ) ) ;
#28866=CARTESIAN_POINT ( 'NONE',  ( 63.98210704970577467, -13.60563849168869943, -8.547981236546295492 ) ) ;
#28905=ORIENTED_EDGE ( 'NONE', *, *, #11962, .T. ) ;
#28911=CARTESIAN_POINT ( 'NONE',  ( -13.61798799253326564, -4.713664127232092937, -7.789724229335226902 ) ) ;
#28914=CARTESIAN_POINT ( 'NONE',  ( 66.08999561209553519, -0.1327762451593314241, -16.39321520033831447 ) ) ;
#28936=VERTEX_POINT ( 'NONE', #8360 ) ;
#28938=CARTESIAN_POINT ( 'NONE',  ( -13.56828337869051104, -4.779084862086333985, -17.89321520033831447 ) ) ;
#28957=AXIS2_PLACEMENT_3D ( 'NONE', #13566, #44809, #33606 ) ;
#28976=FACE_OUTER_BOUND ( 'NONE', #12986, .T. ) ;
#28995=CARTESIAN_POINT ( 'NONE',  ( -12.55641747516330575, -4.307035652475513565, -19.39321520033831447 ) ) ;
#29025=CARTESIAN_POINT ( 'NONE',  ( 3.060777270043529619, -5.064559853354640317, -17.89321520033831447 ) ) ;
#29047=ORIENTED_EDGE ( 'NONE', *, *, #6360, .T. ) ;
#29071=EDGE_CURVE ( 'NONE', #38280, #28936, #6748, .T. ) ;
#29081=CARTESIAN_POINT ( 'NONE',  ( 61.00844462485471098, -13.32659074696883117, -7.515841235333575732 ) ) ;
#29086=CARTESIAN_POINT ( 'NONE',  ( 75.95778847736514194, -3.256761025687008537, -12.39321520033831447 ) ) ;
#29101=CARTESIAN_POINT ( 'NONE',  ( -13.37968822036932615, -5.027311996218202239, -18.18770968788854603 ) ) ;
#29117=CIRCLE ( 'NONE', #35743, 1.499999999999998002 ) ;
#29120=DIRECTION ( 'NONE',  ( 0.000000000000000000, 0.000000000000000000, -1.000000000000000000 ) ) ;
#29121=ORIENTED_EDGE ( 'NONE', *, *, #19491, .F. ) ;
#29130=CARTESIAN_POINT ( 'NONE',  ( 67.94976195724866841, -0.5658009588791762523, -16.39321520033831447 ) ) ;
#29142=CARTESIAN_POINT ( 'NONE',  ( 69.69189222815028018, -41.76310523276638520, -14.39321520033831625 ) ) ;
#29172=( BOUNDED_SURFACE ( )  B_SPLINE_SURFACE ( 3, 2, ( 
 ( #27575, #20728, #3393 ),
 ( #31202, #13880, #27792 ),
 ( #24370, #8160, #39162 ),
 ( #25491, #36183, #21614 ),
 ( #25714, #42594, #4949 ),
 ( #32974, #43038, #11807 ),
 ( #14547, #28911, #1308 ),
 ( #35501, #36401, #15449 ),
 ( #4273, #22065, #7927 ),
 ( #39394, #18862, #18192 ) ),
 .UNSPECIFIED., .F., .F., .F. ) 
 B_SPLINE_SURFACE_WITH_KNOTS ( ( 4, 2, 2, 2, 4 ),
 ( 3, 3 ),
 ( 0.0008626443591432887605, 0.001000512151876073409, 0.001138379944608858057, 0.001276247737341642706, 0.001414115530074427354 ),
 ( 0.000000000000000000, 1.000000000000000000 ),
 .UNSPECIFIED. ) 
 GEOMETRIC_REPRESENTATION_ITEM ( )  RATIONAL_B_SPLINE_SURFACE ( (
 ( 1.000000000000000000, 0.9079001203735632686, 1.000000000000000000),
 ( 1.000000000000000000, 0.9079951794695932943, 1.000000000000000000),
 ( 1.000000000000000000, 0.9016384734332488771, 1.000000000000000000),
 ( 1.000000000000000000, 0.8796635664893247553, 1.000000000000000000),
 ( 1.000000000000000000, 0.8641413844937639865, 1.000000000000000000),
 ( 1.000000000000000000, 0.8276919187008282552, 1.000000000000000000),
 ( 1.000000000000000000, 0.8062482852324636129, 1.000000000000000000),
 ( 1.000000000000000000, 0.7597475340234437491, 1.000000000000000000),
 ( 1.000000000000000000, 0.7345850491789025494, 1.000000000000000000),
 ( 1.000000000000000000, 0.7071067811865467956, 1.000000000000000000) ) ) 
 REPRESENTATION_ITEM ( '' )  SURFACE ( )  );
#29179=EDGE_LOOP ( 'NONE', ( #1620, #31918, #6982, #1683 ) ) ;
#29203=VECTOR ( 'NONE', #15697, 1000.000000000000000 ) ;
#29240=VECTOR ( 'NONE', #44124, 1000.000000000000000 ) ;
#29268=CARTESIAN_POINT ( 'NONE',  ( 62.37505303770993237, -3.555642511118201288, -19.24368838960830885 ) ) ;
#29281=EDGE_CURVE ( 'NONE', #1972, #40326, #36428, .T. ) ;
#29309=CARTESIAN_POINT ( 'NONE',  ( 62.89927913424436667, -13.37923420970709643, -8.047269637219322647 ) ) ;
#29324=CARTESIAN_POINT ( 'NONE',  ( 3.060777270043529619, -5.064559853354640317, -8.893215200338314474 ) ) ;
#29335=EDGE_LOOP ( 'NONE', ( #21405, #312, #27981, #33197 ) ) ;
#29361=VECTOR ( 'NONE', #12214, 1000.000000000000000 ) ;
#29392=( LENGTH_UNIT ( ) NAMED_UNIT ( * ) SI_UNIT ( .MILLI., .METRE. ) );
#29431=CARTESIAN_POINT ( 'NONE',  ( 46.47434218039879283, -17.93412427487546523, -7.393215200338315363 ) ) ;
#29438=CARTESIAN_POINT ( 'NONE',  ( 65.10287265247758626, -0.4742552606671335269, -10.39321520033831625 ) ) ;
#29442=DIRECTION ( 'NONE',  ( -0.9908103287288504424, 0.1352586133457951423, 0.000000000000000000 ) ) ;
#29462=CARTESIAN_POINT ( 'NONE',  ( 65.92808964132663618, -15.33417687497728643, -16.39321520033831447 ) ) ;
#29474=EDGE_CURVE ( 'NONE', #32359, #3982, #22433, .T. ) ;
#29475=ORIENTED_EDGE ( 'NONE', *, *, #30899, .F. ) ;
#29503=ORIENTED_EDGE ( 'NONE', *, *, #15842, .F. ) ;
#29511=EDGE_CURVE ( 'NONE', #42460, #17168, #24122, .T. ) ;
#29528=ORIENTED_EDGE ( 'NONE', *, *, #25373, .F. ) ;
#29533=CARTESIAN_POINT ( 'NONE',  ( 65.25964473381483799, -0.4011607976803650000, -10.39321520033831447 ) ) ;
#29534=CARTESIAN_POINT ( 'NONE',  ( -2.287846945405087595, -6.971096200682639576, -19.14905881027154422 ) ) ;
#29535=CARTESIAN_POINT ( 'NONE',  ( 62.31172044813433075, -14.51131609691315383, -9.168783104843154064 ) ) ;
#29540=CARTESIAN_POINT ( 'NONE',  ( 65.52069343109694444, -15.46830775796534319, -10.39321520033831625 ) ) ;
#29563=AXIS2_PLACEMENT_3D ( 'NONE', #28056, #18008, #7515 ) ;
#29573=EDGE_CURVE ( 'NONE', #7942, #166, #16109, .T. ) ;
#29576=AXIS2_PLACEMENT_3D ( 'NONE', #40996, #3348, #17267 ) ;
#29613=DIRECTION ( 'NONE',  ( 0.1352586133457950590, 0.9908103287288504424, 0.000000000000000000 ) ) ;
#29619=VECTOR ( 'NONE', #40579, 1000.000000000000000 ) ;
#29629=ORIENTED_EDGE ( 'NONE', *, *, #20016, .T. ) ;
#29638=EDGE_CURVE ( 'NONE', #17567, #3982, #19242, .T. ) ;
#29647=ORIENTED_EDGE ( 'NONE', *, *, #29511, .F. ) ;
#29679=CARTESIAN_POINT ( 'NONE',  ( 64.71877406242255404, -15.46959563142843130, -10.63875690036632271 ) ) ;
#29693=AXIS2_PLACEMENT_3D ( 'NONE', #32049, #39124, #1043 ) ;
#29706=ORIENTED_EDGE ( 'NONE', *, *, #42726, .T. ) ;
#29715=DIRECTION ( 'NONE',  ( 0.9908103287288504424, -0.1352586133457950590, 0.000000000000000000 ) ) ;
#29725=ORIENTED_EDGE ( 'NONE', *, *, #19789, .F. ) ;
#29731=ORIENTED_EDGE ( 'NONE', *, *, #32082, .T. ) ;
#29754=CARTESIAN_POINT ( 'NONE',  ( 66.95945348646621653, -0.07477774445813356596, -10.39321520033831270 ) ) ;
#29766=ADVANCED_FACE ( 'NONE', ( #15822 ), #40217, .T. ) ;
#29773=CARTESIAN_POINT ( 'NONE',  ( -13.90346622911597052, -4.337920416975999061, -17.89321520033826474 ) ) ;
#29788=EDGE_CURVE ( 'NONE', #20112, #5874, #35740, .T. ) ;
#29803=CARTESIAN_POINT ( 'NONE',  ( 62.62817532774667484, -3.458832888097430835, -7.587504157255726689 ) ) ;
#29806=CARTESIAN_POINT ( 'NONE',  ( 68.15530245861752690, -1.266379369369464492, -16.39321520033831092 ) ) ;
#29807=DIRECTION ( 'NONE',  ( 0.000000000000000000, 0.000000000000000000, -1.000000000000000000 ) ) ;
#29824=CARTESIAN_POINT ( 'NONE',  ( 80.41643495664496299, -3.865424785743087899, -15.89321520033831447 ) ) ;
#29843=CARTESIAN_POINT ( 'NONE',  ( 2.181596283295915484, -11.50482699009217669, -7.393215200338315363 ) ) ;
#29868=CIRCLE ( 'NONE', #39339, 6.999999999999999112 ) ;
#29945=CARTESIAN_POINT ( 'NONE',  ( 64.59905953672186740, -2.705726756842734559, -18.63794755288801852 ) ) ;
#29964=VERTEX_POINT ( 'NONE', #40675 ) ;
#29971=PLANE ( 'NONE',  #44666 ) ;
#29982=CARTESIAN_POINT ( 'NONE',  ( 66.70735521015549807, -0.06012111411771998981, -10.39321520033831625 ) ) ;
#29990=CARTESIAN_POINT ( 'NONE',  ( 65.92902809793561403, -15.33347626600828839, -10.39321520033831803 ) ) ;
#29999=CARTESIAN_POINT ( 'NONE',  ( -13.43709533753589724, -4.951753300544988967, -8.615451148147142746 ) ) ;
#30001=CARTESIAN_POINT ( 'NONE',  ( -13.59781860028402889, -3.880472447307081740, -18.65072185953338391 ) ) ;
#30025=CARTESIAN_POINT ( 'NONE',  ( 66.56203039180191183, 0.2060721959768717360, -11.55262144894435927 ) ) ;
#30045=DIRECTION ( 'NONE',  ( 0.000000000000000000, 0.000000000000000000, -1.000000000000000000 ) ) ;
#30066=DIRECTION ( 'NONE',  ( 0.1352586133457952255, 0.9908103287288504424, 0.000000000000000000 ) ) ;
#30084=CARTESIAN_POINT ( 'NONE',  ( 9.052690036452151645, -4.182915634381243919, -7.393215200338315363 ) ) ;
#30111=ORIENTED_EDGE ( 'NONE', *, *, #41746, .T. ) ;
#30129=LINE ( 'NONE', #9605, #21288 ) ;
#30146=CARTESIAN_POINT ( 'NONE',  ( 66.09831493924600920, -15.19954166770336990, -16.39321520033831447 ) ) ;
#30172=CARTESIAN_POINT ( 'NONE',  ( 64.40214619852623912, -2.780995199376929516, -18.71258234879876881 ) ) ;
#30177=CARTESIAN_POINT ( 'NONE',  ( -2.128438283008827092, -6.923168977537326185, -7.764336790352773576 ) ) ;
#30213=CARTESIAN_POINT ( 'NONE',  ( -2.674541079949086519, -7.087030491801339593, -19.34356310333839701 ) ) ;
#30229=DIRECTION ( 'NONE',  ( -0.9908103287288505534, 0.1352586133457950590, 0.000000000000000000 ) ) ;
#30238=VECTOR ( 'NONE', #3222, 1000.000000000000000 ) ;
#30249=VERTEX_POINT ( 'NONE', #10207 ) ;
#30280=EDGE_LOOP ( 'NONE', ( #17145, #44447, #37084, #30587 ) ) ;
#30356=VECTOR ( 'NONE', #12123, 1000.000000000000000 ) ;
#30359=ORIENTED_EDGE ( 'NONE', *, *, #23670, .T. ) ;
#30380=LINE ( 'NONE', #37196, #7273 ) ;
#30388=VECTOR ( 'NONE', #11468, 1000.000000000000000 ) ;
#30400=LINE ( 'NONE', #41359, #32795 ) ;
#30402=CARTESIAN_POINT ( 'NONE',  ( -3.075987277002964593, -7.207016596002466358, -7.393215200338315363 ) ) ;
#30412=AXIS2_PLACEMENT_3D ( 'NONE', #29086, #36363, #19051 ) ;
#30427=CARTESIAN_POINT ( 'NONE',  ( 27.57768543387103222, -14.97172645945875935, -17.89321520033831447 ) ) ;
#30433=EDGE_LOOP ( 'NONE', ( #43146, #21991, #31909, #1228 ) ) ;
#30437=CARTESIAN_POINT ( 'NONE',  ( 67.90958954586700713, -0.5136061671847661492, -10.39321520033831625 ) ) ;
#30458=DIRECTION ( 'NONE',  ( 0.1352586133457950590, 0.9908103287288504424, 0.000000000000000000 ) ) ;
#30504=VERTEX_POINT ( 'NONE', #36982 ) ;
#30507=DIRECTION ( 'NONE',  ( -0.9908103287288504424, 0.1352586133457950313, 0.000000000000000000 ) ) ;
#30511=DIRECTION ( 'NONE',  ( 0.9908103287288504424, -0.1352586133457950590, 0.000000000000000000 ) ) ;
#30530=ORIENTED_EDGE ( 'NONE', *, *, #4240, .T. ) ;
#30534=CARTESIAN_POINT ( 'NONE',  ( 66.50565249108366572, -35.53029877516337365, -7.393215200338315363 ) ) ;
#30565=ORIENTED_EDGE ( 'NONE', *, *, #31406, .F. ) ;
#30587=ORIENTED_EDGE ( 'NONE', *, *, #26449, .F. ) ;
#30588=VECTOR ( 'NONE', #6796, 1000.000000000000000 ) ;
#30594=EDGE_CURVE ( 'NONE', #39376, #4486, #20365, .T. ) ;
#30621=ADVANCED_FACE ( 'NONE', ( #27432 ), #41890, .T. ) ;
#30626=ORIENTED_EDGE ( 'NONE', *, *, #9988, .F. ) ;
#30644=AXIS2_PLACEMENT_3D ( 'NONE', #44093, #37454, #33799 ) ;
#30651=CARTESIAN_POINT ( 'NONE',  ( 59.41474631770697812, -13.68180984308303039, -7.393215200338313586 ) ) ;
#30652=CARTESIAN_POINT ( 'NONE',  ( 61.41196271890139258, -3.923926642757838756, -7.421452497510491852 ) ) ;
#30656=DIRECTION ( 'NONE',  ( 0.1352586133457950590, 0.9908103287288504424, 0.000000000000000000 ) ) ;
#30682=FACE_OUTER_BOUND ( 'NONE', #11025, .T. ) ;
#30701=CARTESIAN_POINT ( 'NONE',  ( 80.91184012100937650, -3.933054092416038650, -10.89321520033831447 ) ) ;
#30706=DIRECTION ( 'NONE',  ( -0.9908103287288504424, 0.1352586133457950590, 0.000000000000000000 ) ) ;
#30715=VECTOR ( 'NONE', #21698, 1000.000000000000000 ) ;
#30739=ORIENTED_EDGE ( 'NONE', *, *, #4911, .F. ) ;
#30751=AXIS2_PLACEMENT_3D ( 'NONE', #4297, #38068, #28490 ) ;
#30765=AXIS2_PLACEMENT_3D ( 'NONE', #44491, #10729, #6859 ) ;
#30780=AXIS2_PLACEMENT_3D ( 'NONE', #33937, #16180, #9334 ) ;
#30804=AXIS2_PLACEMENT_3D ( 'NONE', #21527, #4638, #31333 ) ;
#30819=FACE_OUTER_BOUND ( 'NONE', #24306, .T. ) ;
#30883=ORIENTED_EDGE ( 'NONE', *, *, #11364, .T. ) ;
#30899=EDGE_CURVE ( 'NONE', #23226, #6624, #27875, .T. ) ;
#30912=ORIENTED_EDGE ( 'NONE', *, *, #17126, .F. ) ;
#30918=SHAPE_REPRESENTATION ( 'Body4', ( #12375 ), #19397 ) ;
#30941=FACE_OUTER_BOUND ( 'NONE', #8376, .T. ) ;
#30943=ORIENTED_EDGE ( 'NONE', *, *, #26428, .F. ) ;
#30979=CARTESIAN_POINT ( 'NONE',  ( -13.56828337869051104, -4.779084862086335761, -17.89321520033831447 ) ) ;
#30981=AXIS2_PLACEMENT_3D ( 'NONE', #20788, #3455, #17372 ) ;
#31005=ORIENTED_EDGE ( 'NONE', *, *, #34499, .T. ) ;
#31011=VERTEX_POINT ( 'NONE', #29431 ) ;
#31027=CARTESIAN_POINT ( 'NONE',  ( 41.72636039845269096, -11.37347657059392070, -19.39321520033831447 ) ) ;
#31045=DIRECTION ( 'NONE',  ( 0.000000000000000000, 0.000000000000000000, 1.000000000000000000 ) ) ;
#31048=TOROIDAL_SURFACE ( 'NONE', #3388, 5.500000000000000000, 0.5000000000000000000 ) ;
#31065=DIRECTION ( 'NONE',  ( -0.1352586133457953366, -0.9908103287288504424, 0.000000000000000000 ) ) ;
#31068=FACE_OUTER_BOUND ( 'NONE', #23979, .T. ) ;
#31071=AXIS2_PLACEMENT_3D ( 'NONE', #26246, #43127, #8472 ) ;
#31093=CARTESIAN_POINT ( 'NONE',  ( 59.78685257969296174, -14.81377569729348664, -7.401628058557651713 ) ) ;
#31094=CARTESIAN_POINT ( 'NONE',  ( 62.62390430415688769, -3.460464904265341701, -7.586702879152205092 ) ) ;
#31096=CIRCLE ( 'NONE', #39853, 6.999999999999999112 ) ;
#31110=DIRECTION ( 'NONE',  ( -0.1352586133457950590, -0.9908103287288504424, 0.000000000000000000 ) ) ;
#31116=CARTESIAN_POINT ( 'NONE',  ( 61.63318325272354770, -19.46990085680238636, -10.39321520033831625 ) ) ;
#31148=CARTESIAN_POINT ( 'NONE',  ( 71.31713442278437753, 2.423123680056944007, -10.89321520033831447 ) ) ;
#31150=EDGE_CURVE ( 'NONE', #43799, #2987, #15982, .T. ) ;
#31151=CARTESIAN_POINT ( 'NONE',  ( 61.13536639111517701, -12.48752525818348502, -17.20977388067641556 ) ) ;
#31183=ORIENTED_EDGE ( 'NONE', *, *, #37847, .T. ) ;
#31202=CARTESIAN_POINT ( 'NONE',  ( -13.56828338283517787, -4.779084856631165223, -8.846726502787863211 ) ) ;
#31215=ORIENTED_EDGE ( 'NONE', *, *, #37812, .F. ) ;
#31226=CARTESIAN_POINT ( 'NONE',  ( 9.052690036452151645, -4.182915634381243919, -17.89321520033831447 ) ) ;
#31259=FACE_OUTER_BOUND ( 'NONE', #29179, .T. ) ;
#31301=DIRECTION ( 'NONE',  ( 0.000000000000000000, 0.000000000000000000, 1.000000000000000000 ) ) ;
#31309=DIRECTION ( 'NONE',  ( -0.9908103287288505534, 0.1352586133457950868, 0.000000000000000000 ) ) ;
#31333=DIRECTION ( 'NONE',  ( 0.9908103287288504424, -0.1352586133457950868, 0.000000000000000000 ) ) ;
#31335=CARTESIAN_POINT ( 'NONE',  ( 35.90261398037149121, 14.17005867477686820, -18.19321520033831519 ) ) ;
#31347=VERTEX_POINT ( 'NONE', #12567 ) ;
#31366=CARTESIAN_POINT ( 'NONE',  ( 64.24243542014160369, -41.01918285936451269, -15.89321520033831447 ) ) ;
#31368=CARTESIAN_POINT ( 'NONE',  ( 63.78293339202748058, -12.80721147464382881, -16.09572056279317920 ) ) ;
#31373=VECTOR ( 'NONE', #4525, 1000.000000000000000 ) ;
#31383=FACE_OUTER_BOUND ( 'NONE', #18845, .T. ) ;
#31406=EDGE_CURVE ( 'NONE', #39715, #32385, #37154, .T. ) ;
#31425=EDGE_CURVE ( 'NONE', #511, #27420, #5964, .T. ) ;
#31438=AXIS2_PLACEMENT_3D ( 'NONE', #4153, #31961, #14424 ) ;
#31445=CARTESIAN_POINT ( 'NONE',  ( 63.69952534844841807, -14.91276996408597810, -16.69749735386625744 ) ) ;
#31458=CYLINDRICAL_SURFACE ( 'NONE', #18409, 4.999999999999998224 ) ;
#31490=ORIENTED_EDGE ( 'NONE', *, *, #17797, .F. ) ;
#31521=CARTESIAN_POINT ( 'NONE',  ( -12.36826994950263625, -4.374949827406447334, -18.19321520033831519 ) ) ;
#31558=CARTESIAN_POINT ( 'NONE',  ( 77.44400397045842510, -3.459648945705700473, -7.147228641687434880 ) ) ;
#31560=VERTEX_POINT ( 'NONE', #10269 ) ;
#31593=CARTESIAN_POINT ( 'NONE',  ( 59.73260846536648927, -12.72599336462991282, -17.39039534737584347 ) ) ;
#31625=CARTESIAN_POINT ( 'NONE',  ( 61.94466824697356344, -46.76115691171892053, -10.39321520033831625 ) ) ;
#31639=VERTEX_POINT ( 'NONE', #18219 ) ;
#31654=DIRECTION ( 'NONE',  ( 0.9908103287288502203, -0.1352586133457969741, 0.000000000000000000 ) ) ;
#31667=CARTESIAN_POINT ( 'NONE',  ( 60.96715249881023624, -14.49348130257909162, -18.08530754977647703 ) ) ;
#31670=DIRECTION ( 'NONE',  ( -0.9498278979187092519, -0.3127730236694430399, 0.000000000000000000 ) ) ;
#31701=EDGE_CURVE ( 'NONE', #25838, #31560, #27825, .T. ) ;
#31703=CARTESIAN_POINT ( 'NONE',  ( 71.31713442278437753, 2.423123680056944007, -15.89321520033831447 ) ) ;
#31726=AXIS2_PLACEMENT_3D ( 'NONE', #9680, #17418, #31309 ) ;
#31737=CYLINDRICAL_SURFACE ( 'NONE', #810, 5.000000000000000888 ) ;
#31742=VERTEX_POINT ( 'NONE', #28030 ) ;
#31757=VECTOR ( 'NONE', #14893, 1000.000000000000114 ) ;
#31759=ORIENTED_EDGE ( 'NONE', *, *, #35709, .T. ) ;
#31760=FACE_OUTER_BOUND ( 'NONE', #38369, .T. ) ;
#31781=FACE_OUTER_BOUND ( 'NONE', #37263, .T. ) ;
#31783=ADVANCED_FACE ( 'NONE', ( #12613 ), #26516, .T. ) ;
#31788=CARTESIAN_POINT ( 'NONE',  ( 65.01991922978720595, -13.34372148804275149, -11.74794487108197849 ) ) ;
#31797=AXIS2_PLACEMENT_3D ( 'NONE', #20950, #25037, #28019 ) ;
#31808=CARTESIAN_POINT ( 'NONE',  ( 62.16677121968579200, -14.49431128105087829, -9.102658187437317139 ) ) ;
#31819=CARTESIAN_POINT ( 'NONE',  ( -1.307700928565892706, -16.07486664983353819, -19.39321520033831447 ) ) ;
#31820=DIRECTION ( 'NONE',  ( 0.6049664196031392382, -0.7962509850245451659, 0.000000000000000000 ) ) ;
#31824=B_SPLINE_CURVE_WITH_KNOTS ( 'NONE', 3,
 ( #9240, #29533, #43449, #26111, #40017, #22686, #26341, #19719, #15858, #1706, #40704, #29982, #37256, #8782, #6029, #22914, #29754, #19951, #36806, #36585, #16078, #43900, #5800, #5360, #5575, #40480, #26567, #19498, #23375, #19277, #30437, #12898, #33604, #13117, #33377, #2148, #23149 ),
 .UNSPECIFIED., .F., .F.,
 ( 4, 1, 1, 1, 1, 2, 2, 1, 1, 1, 1, 2, 2, 1, 1, 1, 2, 2, 1, 1, 2, 2, 2, 2, 4 ),
 ( 0.000000000000000000, 0.1250000000000005274, 0.1875000000000007772, 0.2187499999999955314, 0.2343749999999929223, 0.2421874999999915901, 0.2499999999999902855, 0.3749999999999692468, 0.4374999999999587552, 0.4687499999999535372, 0.4843749999999566458, 0.4921874999999523714, 0.4999999999999481526, 0.5624999999999441558, 0.5937499999999422684, 0.6093749999999412692, 0.6171874999999459321, 0.6249999999999507061, 0.6874999999999606981, 0.7187499999999656941, 0.7343749999999725775, 0.7499999999999793499, 0.8124999999999845679, 0.8749999999999896749, 1.000000000000000000 ),
 .UNSPECIFIED. ) ;
#31828=ORIENTED_EDGE ( 'NONE', *, *, #38036, .T. ) ;
#31861=B_SPLINE_CURVE_WITH_KNOTS ( 'NONE', 3,
 ( #944, #15084, #11664, #39021, #4584, #42455, #15303, #14633, #712, #7561, #42009, #14863, #21920, #24669, #28772, #11448 ),
 .UNSPECIFIED., .F., .F.,
 ( 4, 2, 2, 2, 2, 2, 2, 4 ),
 ( 1.734723475976806902E-18, 0.0009594866571110036938, 0.001918973314222005653, 0.002878459971333007829, 0.003837946628444009571, 0.004797433285555011313, 0.005756919942666013923, 0.007675893256888017407 ),
 .UNSPECIFIED. ) ;
#31894=CARTESIAN_POINT ( 'NONE',  ( 63.51875845105345064, -14.83467802062719798, -16.85055330987278666 ) ) ;
#31897=ORIENTED_EDGE ( 'NONE', *, *, #35709, .F. ) ;
#31909=ORIENTED_EDGE ( 'NONE', *, *, #30899, .T. ) ;
#31912=CARTESIAN_POINT ( 'NONE',  ( 59.90552009294155766, -2.897503654462286971, -19.39321520033830737 ) ) ;
#31918=ORIENTED_EDGE ( 'NONE', *, *, #4258, .F. ) ;
#31947=CARTESIAN_POINT ( 'NONE',  ( -13.74785857260074096, -3.813629379304071421, -18.29023369286690581 ) ) ;
#31961=DIRECTION ( 'NONE',  ( 0.000000000000000000, 0.000000000000000000, -1.000000000000000000 ) ) ;
#31979=DIRECTION ( 'NONE',  ( -0.9908103287288504424, 0.1352586133457952811, 0.000000000000000000 ) ) ;
#32005=CARTESIAN_POINT ( 'NONE',  ( 58.92639935879823554, -16.07256461744605147, -19.39321520033831447 ) ) ;
#32008=CARTESIAN_POINT ( 'NONE',  ( 65.02437422720751670, -13.34618800689889362, -11.75271837916926820 ) ) ;
#32034=CIRCLE ( 'NONE', #12407, 1.199999999999999734 ) ;
#32035=DIRECTION ( 'NONE',  ( 0.1352586133457950590, 0.9908103287288504424, 0.000000000000000000 ) ) ;
#32042=CARTESIAN_POINT ( 'NONE',  ( 0.04488520489200759078, -6.166763362545027327, -18.19321520033831519 ) ) ;
#32044=CARTESIAN_POINT ( 'NONE',  ( 65.91876108126248823, -14.44801200876193192, -9.970851920820145153 ) ) ;
#32049=CARTESIAN_POINT ( 'NONE',  ( 54.86886719809545809, -45.79521720516596872, -9.393215200338314474 ) ) ;
#32082=EDGE_CURVE ( 'NONE', #36383, #15954, #1632, .T. ) ;
#32109=CARTESIAN_POINT ( 'NONE',  ( -3.429934629567074733, -4.841764211284793618, -17.89321520033831447 ) ) ;
#32111=CARTESIAN_POINT ( 'NONE',  ( -1.932019669644797988, -4.762702382056356321, -8.893215200338314474 ) ) ;
#32117=CARTESIAN_POINT ( 'NONE',  ( 62.99192496234383043, -14.62834943820164746, -18.63369276689623533 ) ) ;
#32127=( NAMED_UNIT ( * ) PLANE_ANGLE_UNIT ( ) SI_UNIT ( $, .RADIAN. ) );
#32137=CARTESIAN_POINT ( 'NONE',  ( 61.35525772184064408, -2.221568293060733001, -19.50743695395307853 ) ) ;
#32146=CARTESIAN_POINT ( 'NONE',  ( 74.47157298427187300, -3.053873105668316601, -10.39321520033831625 ) ) ;
#32175=CARTESIAN_POINT ( 'NONE',  ( -12.73631100612642797, -4.238385078766282454, -19.35607154375884775 ) ) ;
#32179=VERTEX_POINT ( 'NONE', #22083 ) ;
#32180=DIRECTION ( 'NONE',  ( 0.7962509850245486076, 0.6049664196031347974, 0.000000000000000000 ) ) ;
#32187=EDGE_LOOP ( 'NONE', ( #17816, #42366, #41588, #43418 ) ) ;
#32192=LINE ( 'NONE', #39720, #30388 ) ;
#32196=EDGE_LOOP ( 'NONE', ( #20416, #40631, #34601, #9336 ) ) ;
#32214=CIRCLE ( 'NONE', #41005, 1.499999999999998002 ) ;
#32216=AXIS2_PLACEMENT_3D ( 'NONE', #6279, #20199, #37961 ) ;
#32235=CARTESIAN_POINT ( 'NONE',  ( 63.22841645929758414, -12.65390981026857453, -10.35299945512634245 ) ) ;
#32270=CARTESIAN_POINT ( 'NONE',  ( 65.71141733757100667, -16.34216531378293524, -9.991044251572791524 ) ) ;
#32314=AXIS2_PLACEMENT_3D ( 'NONE', #10524, #24424, #34665 ) ;
#32319=CARTESIAN_POINT ( 'NONE',  ( 64.37076103624345080, -2.792960894985629938, -8.058217223812896179 ) ) ;
#32344=CARTESIAN_POINT ( 'NONE',  ( 63.19915535949495222, -13.42640250087169385, -18.61752652045166911 ) ) ;
#32354=SURFACE_STYLE_FILL_AREA ( #25975 ) ;
#32356=DIRECTION ( 'NONE',  ( 0.9908103287288504424, -0.1352586133457951423, 0.000000000000000000 ) ) ;
#32359=VERTEX_POINT ( 'NONE', #32805 ) ;
#32377=DIRECTION ( 'NONE',  ( 0.000000000000000000, 0.000000000000000000, -1.000000000000000000 ) ) ;
#32378=CYLINDRICAL_SURFACE ( 'NONE', #44146, 0.4999999999999996669 ) ;
#32385=VERTEX_POINT ( 'NONE', #28740 ) ;
#32411=ORIENTED_EDGE ( 'NONE', *, *, #40657, .F. ) ;
#32417=ORIENTED_EDGE ( 'NONE', *, *, #37255, .T. ) ;
#32432=EDGE_CURVE ( 'NONE', #24584, #31011, #38035, .T. ) ;
#32462=DIRECTION ( 'NONE',  ( 0.000000000000000000, 0.000000000000000000, 1.000000000000000000 ) ) ;
#32472=AXIS2_PLACEMENT_3D ( 'NONE', #18466, #28279, #14817 ) ;
#32485=CARTESIAN_POINT ( 'NONE',  ( -12.73765092793578191, -4.237858357736757675, -7.430846270786123142 ) ) ;
#32489=CARTESIAN_POINT ( 'NONE',  ( 68.56885555382550024, -20.41671115022302274, -14.39321520033831625 ) ) ;
#32490=CARTESIAN_POINT ( 'NONE',  ( 60.11760374155739584, -14.70486118635414385, -7.429569208445769846 ) ) ;
#32507=CARTESIAN_POINT ( 'NONE',  ( -13.55920938158181599, -4.791027969838746792, -8.800393969189304499 ) ) ;
#32531=EDGE_CURVE ( 'NONE', #27501, #17020, #5288, .T. ) ;
#32534=EDGE_CURVE ( 'NONE', #42200, #16463, #11124, .T. ) ;
#32545=CARTESIAN_POINT ( 'NONE',  ( 78.93021946355167984, -3.662536865724447921, -14.39321520033831625 ) ) ;
#32549=ADVANCED_FACE ( 'NONE', ( #33255 ), #22763, .T. ) ;
#32555=EDGE_CURVE ( 'NONE', #11788, #16463, #6739, .T. ) ;
#32566=CARTESIAN_POINT ( 'NONE',  ( -13.43670958668108462, -4.952261022111287936, -18.17119155822705778 ) ) ;
#32583=CARTESIAN_POINT ( 'NONE',  ( 31.16203868753470019, 11.28474725185576055, -8.893215200338314474 ) ) ;
#32584=ORIENTED_EDGE ( 'NONE', *, *, #14765, .F. ) ;
#32650=ORIENTED_EDGE ( 'NONE', *, *, #26741, .F. ) ;
#32658=DIRECTION ( 'NONE',  ( 0.000000000000000000, 0.000000000000000000, 1.000000000000000000 ) ) ;
#32659=EDGE_LOOP ( 'NONE', ( #4885, #4548, #38083, #14935 ) ) ;
#32683=CARTESIAN_POINT ( 'NONE',  ( 78.93021946355167984, -3.662536865724447921, -19.39321520033831447 ) ) ;
#32690=EDGE_CURVE ( 'NONE', #35231, #1795, #24149, .T. ) ;
#32709=CARTESIAN_POINT ( 'NONE',  ( -2.040426804217055246, -6.896677610160479865, -18.93444115535162453 ) ) ;
#32710=CARTESIAN_POINT ( 'NONE',  ( 61.93156847455978919, -13.30602482174417389, -7.732832247245597479 ) ) ;
#32716=CARTESIAN_POINT ( 'NONE',  ( 69.69189222815028018, -41.76310523276638520, -10.89321520033831447 ) ) ;
#32757=CARTESIAN_POINT ( 'NONE',  ( 68.15795393973013461, -1.183743427963408701, -16.39321520033831447 ) ) ;
#32795=VECTOR ( 'NONE', #44322, 1000.000000000000114 ) ;
#32797=CARTESIAN_POINT ( 'NONE',  ( 64.66964420208745423, -0.6762465888536760561, -16.74452531359828100 ) ) ;
#32799=EDGE_CURVE ( 'NONE', #23633, #37929, #10024, .T. ) ;
#32805=CARTESIAN_POINT ( 'NONE',  ( 78.93021946355167984, -3.662536865724447921, -14.39321520033831625 ) ) ;
#32810=CARTESIAN_POINT ( 'NONE',  ( 74.47157298427187300, -3.053873105668316601, -16.39321520033831447 ) ) ;
#32825=CARTESIAN_POINT ( 'NONE',  ( -1.307700928565892706, -16.07486664983353819, -8.593215200338315540 ) ) ;
#32827=EDGE_CURVE ( 'NONE', #13151, #1972, #20944, .T. ) ;
#32837=EDGE_CURVE ( 'NONE', #16463, #12130, #6004, .T. ) ;
#32864=B_SPLINE_CURVE_WITH_KNOTS ( 'NONE', 3,
 ( #20681, #31593, #34558, #21337, #7647, #21562, #24541, #3342, #31151, #20901, #10637, #362, #45071, #13831, #3996, #17918, #27746, #10419, #24326, #34775, #3557, #17471, #31368, #140, #41876, #21788, #36127, #36578, #39786, #43215, #43442, #22680, #22231, #15620, #8332, #5354, #25663, #11754, #18593, #26104, #25884, #36350, #8555 ),
 .UNSPECIFIED., .F., .F.,
 ( 4, 2, 2, 1, 2, 2, 2, 2, 1, 1, 2, 2, 2, 2, 1, 1, 1, 2, 2, 2, 1, 1, 1, 2, 2, 4 ),
 ( 0.000000000000000000, 0.1249999999999658051, 0.1874999999999473199, 0.2187499999999395206, 0.2343749999999356071, 0.2499999999999317213, 0.3749999999998905320, 0.4374999999998702149, 0.4687499999998600564, 0.4843749999998577249, 0.4921874999998566147, 0.4999999999998554490, 0.6249999999998734346, 0.6874999999998797628, 0.7187499999998828715, 0.7343749999998823164, 0.7421874999998844258, 0.7460937499998878675, 0.7499999999998911981, 0.8124999999999091838, 0.8437499999999180655, 0.8593749999999241718, 0.8671874999999273914, 0.8710937499999307221, 0.8749999999999339417, 1.000000000000000000 ),
 .UNSPECIFIED. ) ;
#32868=DIRECTION ( 'NONE',  ( -1.000000000000000000, 0.000000000000000000, 0.000000000000000000 ) ) ;
#32891=CARTESIAN_POINT ( 'NONE',  ( -2.105898499509477162, -6.916383580925556274, -7.785241425804852788 ) ) ;
#32897=DIRECTION ( 'NONE',  ( 0.000000000000000000, 0.000000000000000000, -1.000000000000000000 ) ) ;
#32904=AXIS2_PLACEMENT_3D ( 'NONE', #2786, #20961, #7050 ) ;
#32933=CARTESIAN_POINT ( 'NONE',  ( 64.76452260854006227, -13.87123648633732031, -9.027055449389660424 ) ) ;
#32954=LINE ( 'NONE', #15429, #27231 ) ;
#32957=VECTOR ( 'NONE', #2979, 1000.000000000000000 ) ;
#32974=CARTESIAN_POINT ( 'NONE',  ( -13.46067391278434400, -4.920719406499494575, -8.640382031922472450 ) ) ;
#32975=CARTESIAN_POINT ( 'NONE',  ( 46.84966980880212617, -19.07391775237791620, -18.19321520033831519 ) ) ;
#32977=CARTESIAN_POINT ( 'NONE',  ( 65.41915898433887833, -0.3267878074046857706, -16.39321520033831447 ) ) ;
#32983=AXIS2_PLACEMENT_3D ( 'NONE', #42218, #41166, #27023 ) ;
#33024=DIRECTION ( 'NONE',  ( -1.000000000000000000, 0.000000000000000000, 0.000000000000000000 ) ) ;
#33044=ORIENTED_EDGE ( 'NONE', *, *, #5695, .F. ) ;
#33081=ADVANCED_FACE ( 'NONE', ( #33417 ), #15196, .T. ) ;
#33170=CARTESIAN_POINT ( 'NONE',  ( 41.72636039845269096, -11.37347657059392070, -17.89321520033831447 ) ) ;
#33173=CARTESIAN_POINT ( 'NONE',  ( -13.90346626007465147, -4.337920376228211694, -18.05487786542591166 ) ) ;
#33197=ORIENTED_EDGE ( 'NONE', *, *, #1035, .T. ) ;
#33206=CARTESIAN_POINT ( 'NONE',  ( 68.13072346129467860, -0.9465212610118308723, -16.39321520033831447 ) ) ;
#33232=VERTEX_POINT ( 'NONE', #3989 ) ;
#33239=AXIS2_PLACEMENT_3D ( 'NONE', #9478, #41629, #17010 ) ;
#33240=ORIENTED_EDGE ( 'NONE', *, *, #25993, .F. ) ;
#33252=VERTEX_POINT ( 'NONE', #24976 ) ;
#33255=FACE_OUTER_BOUND ( 'NONE', #20437, .T. ) ;
#33316=VECTOR ( 'NONE', #3568, 1000.000000000000000 ) ;
#33335=CARTESIAN_POINT ( 'NONE',  ( 63.88436160695720645, -2.978941093719386757, -18.88846529135332020 ) ) ;
#33339=CARTESIAN_POINT ( 'NONE',  ( -2.667303743122483528, -7.084803291745695120, -7.454506892862497125 ) ) ;
#33363=EDGE_CURVE ( 'NONE', #31639, #32385, #20938, .T. ) ;
#33365=CARTESIAN_POINT ( 'NONE',  ( 67.19031194842951038, -1.707697914625855296, -12.39321520033831447 ) ) ;
#33377=CARTESIAN_POINT ( 'NONE',  ( 68.15423470349523427, -1.018375365046214620, -10.39321520033831803 ) ) ;
#33384=CARTESIAN_POINT ( 'NONE',  ( 66.09777208604641885, -15.19992928687715761, -10.39321520033831625 ) ) ;
#33394=CARTESIAN_POINT ( 'NONE',  ( -13.40747672045794481, -4.990737039574640654, -19.30361446747916787 ) ) ;
#33417=FACE_OUTER_BOUND ( 'NONE', #22835, .T. ) ;
#33421=CARTESIAN_POINT ( 'NONE',  ( 68.08131077845983725, -0.7911846277411741513, -16.39321520033831447 ) ) ;
#33431=ORIENTED_EDGE ( 'NONE', *, *, #31150, .T. ) ;
#33451=ORIENTED_EDGE ( 'NONE', *, *, #522, .T. ) ;
#33460=CIRCLE ( 'NONE', #18930, 35.00000000000000000 ) ;
#33478=EDGE_CURVE ( 'NONE', #28936, #26194, #44912, .T. ) ;
#33485=DIRECTION ( 'NONE',  ( 0.000000000000000000, 0.000000000000000000, -1.000000000000000000 ) ) ;
#33508=CARTESIAN_POINT ( 'NONE',  ( 74.64594387179452895, -42.43939829949535181, -16.39321520033831447 ) ) ;
#33548=DIRECTION ( 'NONE',  ( -4.625929269271481378E-15, 1.156482317317870344E-15, 1.000000000000000000 ) ) ;
#33604=CARTESIAN_POINT ( 'NONE',  ( 68.04603467680756523, -0.7145533168453219730, -10.39321520033831980 ) ) ;
#33606=DIRECTION ( 'NONE',  ( -0.9908103287288504424, 0.1352586133457950590, 0.000000000000000000 ) ) ;
#33629=EDGE_CURVE ( 'NONE', #20112, #24167, #21333, .T. ) ;
#33654=ADVANCED_FACE ( 'NONE', ( #43886 ), #29971, .F. ) ;
#33711=AXIS2_PLACEMENT_3D ( 'NONE', #764, #18783, #7612 ) ;
#33717=CARTESIAN_POINT ( 'NONE',  ( 68.14371629974728251, -1.351251493923715685, -16.39321520033831447 ) ) ;
#33730=ORIENTED_EDGE ( 'NONE', *, *, #857, .T. ) ;
#33748=CARTESIAN_POINT ( 'NONE',  ( 69.69189222815028018, -41.76310523276638520, -10.39321520033831625 ) ) ;
#33750=AXIS2_PLACEMENT_3D ( 'NONE', #23748, #27613, #37857 ) ;
#33773=CARTESIAN_POINT ( 'NONE',  ( 69.69189222815028018, -41.76310523276638520, -16.39321520033831447 ) ) ;
#33799=DIRECTION ( 'NONE',  ( 0.1352586133457981954, 0.9908103287288499983, 0.000000000000000000 ) ) ;
#33801=CARTESIAN_POINT ( 'NONE',  ( -2.065049201022524539, -6.904086573307711916, -7.826012730671462414 ) ) ;
#33812=AXIS2_PLACEMENT_3D ( 'NONE', #27797, #41710, #10475 ) ;
#33827=CARTESIAN_POINT ( 'NONE',  ( 59.95220766929363521, -14.75932518950456185, -7.413731407758326952 ) ) ;
#33841=CARTESIAN_POINT ( 'NONE',  ( -2.517858533981217395, -7.040069435492971373, -19.27574816075459552 ) ) ;
#33846=DIRECTION ( 'NONE',  ( 0.000000000000000000, 0.000000000000000000, 1.000000000000000000 ) ) ;
#33882=CARTESIAN_POINT ( 'NONE',  ( 66.58723489636778936, -20.14619392353143112, -15.89321520033831447 ) ) ;
#33887=EDGE_CURVE ( 'NONE', #10182, #2987, #42933, .T. ) ;
#33937=CARTESIAN_POINT ( 'NONE',  ( 75.95778847736514194, -3.256761025687008537, -16.39321520033831447 ) ) ;
#33968=VERTEX_POINT ( 'NONE', #24778 ) ;
#33983=DIRECTION ( 'NONE',  ( -0.9908103287288503314, 0.1352586133457956419, 0.000000000000000000 ) ) ;
#33999=ORIENTED_EDGE ( 'NONE', *, *, #5527, .T. ) ;
#34003=FACE_OUTER_BOUND ( 'NONE', #41206, .T. ) ;
#34015=ORIENTED_EDGE ( 'NONE', *, *, #21393, .F. ) ;
#34063=EDGE_CURVE ( 'NONE', #14190, #9071, #5574, .T. ) ;
#34072=DIRECTION ( 'NONE',  ( 0.9908103287288504424, -0.1352586133457950590, 0.000000000000000000 ) ) ;
#34074=DIRECTION ( 'NONE',  ( 0.000000000000000000, 0.000000000000000000, -1.000000000000000000 ) ) ;
#34083=DIRECTION ( 'NONE',  ( -0.9489384314806880161, -0.3124801273375112931, -0.04326688431242012300 ) ) ;
#34096=CARTESIAN_POINT ( 'NONE',  ( -12.36826994950264513, -4.374949827406455327, -8.593215200338315540 ) ) ;
#34111=ORIENTED_EDGE ( 'NONE', *, *, #26685, .T. ) ;
#34124=CYLINDRICAL_SURFACE ( 'NONE', #29576, 1.199999999999999734 ) ;
#34236=CARTESIAN_POINT ( 'NONE',  ( -7.923679509334008664, -5.078949698970065540, -19.39321520033831447 ) ) ;
#34238=ADVANCED_FACE ( 'NONE', ( #2165 ), #20896, .T. ) ;
#34259=ORIENTED_EDGE ( 'NONE', *, *, #4755, .F. ) ;
#34277=CIRCLE ( 'NONE', #9553, 0.5000000000000043299 ) ;
#34284=CARTESIAN_POINT ( 'NONE',  ( 59.92024162955041788, -14.76985142791843053, -8.596615743543749133 ) ) ;
#34304=ADVANCED_FACE ( 'NONE', ( #26581 ), #43448, .T. ) ;
#34336=CARTESIAN_POINT ( 'NONE',  ( 68.14371629974728251, -1.351251493923715685, -10.39321520033831625 ) ) ;
#34345=FACE_OUTER_BOUND ( 'NONE', #29335, .T. ) ;
#34362=ORIENTED_EDGE ( 'NONE', *, *, #13627, .T. ) ;
#34363=CYLINDRICAL_SURFACE ( 'NONE', #10928, 4.999999999999998224 ) ;
#34382=ORIENTED_EDGE ( 'NONE', *, *, #10274, .T. ) ;
#34391=DIRECTION ( 'NONE',  ( 0.9908103287288504424, -0.1352586133457950590, 0.000000000000000000 ) ) ;
#34393=DIRECTION ( 'NONE',  ( 0.000000000000000000, 0.000000000000000000, -1.000000000000000000 ) ) ;
#34417=EDGE_LOOP ( 'NONE', ( #19754, #5184, #22107, #28688 ) ) ;
#34427=EDGE_LOOP ( 'NONE', ( #18217, #22287, #37251, #16981 ) ) ;
#34435=CARTESIAN_POINT ( 'NONE',  ( 59.44377208703740223, -12.82110557137145967, -9.393546723914594665 ) ) ;
#34440=EDGE_LOOP ( 'NONE', ( #37152, #32584, #34382, #10349 ) ) ;
#34443=PLANE ( 'NONE',  #20769 ) ;
#34475=CYLINDRICAL_SURFACE ( 'NONE', #15024, 1.499999999999999556 ) ;
#34484=EDGE_CURVE ( 'NONE', #29964, #36610, #6741, .T. ) ;
#34489=ORIENTED_EDGE ( 'NONE', *, *, #21102, .T. ) ;
#34499=EDGE_CURVE ( 'NONE', #11722, #32385, #8523, .T. ) ;
#34526=DIRECTION ( 'NONE',  ( 0.1352586133457950590, 0.9908103287288504424, 0.000000000000000000 ) ) ;
#34544=( BOUNDED_CURVE ( )  B_SPLINE_CURVE ( 3, ( #23993, #28075, #20565, #38762 ),
 .UNSPECIFIED., .F., .F. ) 
 B_SPLINE_CURVE_WITH_KNOTS ( ( 4, 4 ),
 ( 4.712388980384689674, 4.760535684117931154 ),
 .UNSPECIFIED. ) 
 CURVE ( )  GEOMETRIC_REPRESENTATION_ITEM ( )  RATIONAL_B_SPLINE_CURVE ( ( 1.000000000000000000, 0.9998068339056410680, 0.9998068339056410680, 1.000000000000000000 ) ) 
 REPRESENTATION_ITEM ( '' )  );
#34545=AXIS2_PLACEMENT_3D ( 'NONE', #6269, #34074, #26344 ) ;
#34552=CARTESIAN_POINT ( 'NONE',  ( 60.53937939559665438, -4.256997083809236138, -7.393215200338315363 ) ) ;
#34558=CARTESIAN_POINT ( 'NONE',  ( 60.02532325032445470, -12.65039385568375963, -17.37383293601393675 ) ) ;
#34595=DIRECTION ( 'NONE',  ( 0.9908103287288505534, -0.1352586133457951145, 0.000000000000000000 ) ) ;
#34601=ORIENTED_EDGE ( 'NONE', *, *, #18643, .F. ) ;
#34604=CARTESIAN_POINT ( 'NONE',  ( -7.923679509334008664, -5.078949698970065540, -7.393215200338315363 ) ) ;
#34647=ORIENTED_EDGE ( 'NONE', *, *, #21393, .T. ) ;
#34655=PLANE ( 'NONE',  #37111 ) ;
#34665=DIRECTION ( 'NONE',  ( -0.9908103287288503314, 0.1352586133457959749, 0.000000000000000000 ) ) ;
#34676=CIRCLE ( 'NONE', #17934, 5.000000000000005329 ) ;
#34738=AXIS2_PLACEMENT_3D ( 'NONE', #17922, #24547, #809 ) ;
#34775=CARTESIAN_POINT ( 'NONE',  ( 62.89961678332094408, -12.58539693385646885, -16.60389039546696566 ) ) ;
#34779=CARTESIAN_POINT ( 'NONE',  ( 70.47992290675011873, 2.032776587329049978, -10.39321520033831625 ) ) ;
#34782=CYLINDRICAL_SURFACE ( 'NONE', #21443, 6.999999999999999112 ) ;
#34785=LINE ( 'NONE', #20691, #10066 ) ;
#34798=DIRECTION ( 'NONE',  ( -0.9908103287288503314, 0.1352586133457956419, 0.000000000000000000 ) ) ;
#34812=AXIS2_PLACEMENT_3D ( 'NONE', #22319, #12066, #30066 ) ;
#34839=CARTESIAN_POINT ( 'NONE',  ( -13.32377113153209791, -5.100909530930220370, -8.593215200338315540 ) ) ;
#34846=CARTESIAN_POINT ( 'NONE',  ( 61.65122664504198013, -14.46472737607295045, -17.88559175297232784 ) ) ;
#34861=DIRECTION ( 'NONE',  ( -0.9908103287288504424, 0.1352586133457950590, 0.000000000000000000 ) ) ;
#34879=DIRECTION ( 'NONE',  ( 0.9908103287288513306, -0.1352586133457890638, 0.000000000000000000 ) ) ;
#34925=ORIENTED_EDGE ( 'NONE', *, *, #32432, .T. ) ;
#34930=ORIENTED_EDGE ( 'NONE', *, *, #2187, .T. ) ;
#34939=VERTEX_POINT ( 'NONE', #2509 ) ;
#34953=CARTESIAN_POINT ( 'NONE',  ( 62.93082072130040672, -14.63772337389976208, -17.27340791136839471 ) ) ;
#34963=CARTESIAN_POINT ( 'NONE',  ( 75.95778847736514194, -3.256761025687008537, -16.39321520033831447 ) ) ;
#34969=VECTOR ( 'NONE', #9310, 1000.000000000000000 ) ;
#34979=CARTESIAN_POINT ( 'NONE',  ( 63.42533636626423998, -3.154224173321905855, -7.672534579508055508 ) ) ;
#34980=DIRECTION ( 'NONE',  ( 0.000000000000000000, 0.000000000000000000, 1.000000000000000000 ) ) ;
#34986=LINE ( 'NONE', #15623, #43325 ) ;
#35010=CARTESIAN_POINT ( 'NONE',  ( 81.52050388106540879, 0.5255923868638483487, -10.39321520033831625 ) ) ;
#35013=PRODUCT ( 'Body4', 'Body4', '', ( #25923 ) ) ;
#35018=LINE ( 'NONE', #41244, #17024 ) ;
#35051=EDGE_CURVE ( 'NONE', #36955, #43140, #9289, .T. ) ;
#35088=DIRECTION ( 'NONE',  ( 0.000000000000000000, 0.000000000000000000, 1.000000000000000000 ) ) ;
#35103=CARTESIAN_POINT ( 'NONE',  ( -6.962123463324043193, -11.49046785505262136, -8.593215200338315540 ) ) ;
#35129=CARTESIAN_POINT ( 'NONE',  ( -12.36826994950264513, -4.374949827406456215, -19.39321520033831447 ) ) ;
#35141=FACE_OUTER_BOUND ( 'NONE', #8958, .T. ) ;
#35161=ORIENTED_EDGE ( 'NONE', *, *, #40713, .F. ) ;
#35162=AXIS2_PLACEMENT_3D ( 'NONE', #2926, #20715, #34595 ) ;
#35188=ORIENTED_EDGE ( 'NONE', *, *, #30594, .T. ) ;
#35210=ORIENTED_EDGE ( 'NONE', *, *, #18365, .T. ) ;
#35231=VERTEX_POINT ( 'NONE', #37312 ) ;
#35258=VECTOR ( 'NONE', #21619, 1000.000000000000000 ) ;
#35272=( BOUNDED_CURVE ( )  B_SPLINE_CURVE ( 3, ( #3340, #17259, #6987, #31148 ),
 .UNSPECIFIED., .F., .T. ) 
 B_SPLINE_CURVE_WITH_KNOTS ( ( 4, 4 ),
 ( 1.570796326794904996, 3.141592653589790007 ),
 .UNSPECIFIED. ) 
 CURVE ( )  GEOMETRIC_REPRESENTATION_ITEM ( )  RATIONAL_B_SPLINE_CURVE ( ( 1.000000000000000000, 0.8047378541243679351, 0.8047378541243679351, 1.000000000000000000 ) ) 
 REPRESENTATION_ITEM ( '' )  );
#35297=EDGE_CURVE ( 'NONE', #17020, #27501, #13648, .T. ) ;
#35320=ORIENTED_EDGE ( 'NONE', *, *, #22839, .T. ) ;
#35336=PLANE ( 'NONE',  #440 ) ;
#35359=AXIS2_PLACEMENT_3D ( 'NONE', #21054, #25159, #28133 ) ;
#35365=DIRECTION ( 'NONE',  ( 0.6049664196031343533, -0.7962509850245488296, 0.000000000000000000 ) ) ;
#35379=EDGE_CURVE ( 'NONE', #16139, #24584, #20680, .T. ) ;
#35390=AXIS2_PLACEMENT_3D ( 'NONE', #11400, #42188, #17786 ) ;
#35413=CARTESIAN_POINT ( 'NONE',  ( 61.00489063115648491, -4.079117376897293923, -19.39321520033831092 ) ) ;
#35421=CARTESIAN_POINT ( 'NONE',  ( 65.05177286768275735, -13.36142499895917446, -11.78221109098726771 ) ) ;
#35452=VECTOR ( 'NONE', #15227, 1000.000000000000114 ) ;
#35456=CARTESIAN_POINT ( 'NONE',  ( 65.48165112743714644, -14.20078584921842868, -9.574444890468706504 ) ) ;
#35461=FACE_OUTER_BOUND ( 'NONE', #2996, .T. ) ;
#35489=AXIS2_PLACEMENT_3D ( 'NONE', #32716, #15636, #26574 ) ;
#35501=CARTESIAN_POINT ( 'NONE',  ( -13.37983193548284611, -5.027122839767540263, -8.598763672831253757 ) ) ;
#35528=CARTESIAN_POINT ( 'NONE',  ( 74.43213512091445239, -36.61236768192972590, -12.39321520033831447 ) ) ;
#35529=CARTESIAN_POINT ( 'NONE',  ( 62.52445501936042405, -14.54538235898669285, -17.51060916224595942 ) ) ;
#35537=VECTOR ( 'NONE', #7493, 1000.000000000000000 ) ;
#35543=CARTESIAN_POINT ( 'NONE',  ( 27.57768543387103222, -14.97172645945875935, -8.893215200338314474 ) ) ;
#35546=VERTEX_POINT ( 'NONE', #24333 ) ;
#35555=EDGE_LOOP ( 'NONE', ( #34930, #11462, #42613, #39930 ) ) ;
#35581=ADVANCED_FACE ( 'NONE', ( #30941 ), #34782, .T. ) ;
#35608=CARTESIAN_POINT ( 'NONE',  ( 46.84966980880212617, -19.07391775237791620, -8.593215200338315540 ) ) ;
#35622=FACE_OUTER_BOUND ( 'NONE', #39520, .T. ) ;
#35634=CIRCLE ( 'NONE', #5790, 2.999999999999996003 ) ;
#35648=ORIENTED_EDGE ( 'NONE', *, *, #22385, .T. ) ;
#35652=CARTESIAN_POINT ( 'NONE',  ( 64.64935471094501906, -13.15280763797862207, -11.37863450522776532 ) ) ;
#35655=AXIS2_PLACEMENT_3D ( 'NONE', #43387, #1426, #4851 ) ;
#35680=ADVANCED_FACE ( 'NONE', ( #369 ), #13482, .T. ) ;
#35686=CARTESIAN_POINT ( 'NONE',  ( 60.37456837578754687, -13.41642734739171239, -7.433439893800085407 ) ) ;
#35709=EDGE_CURVE ( 'NONE', #11722, #23894, #41453, .T. ) ;
#35711=ORIENTED_EDGE ( 'NONE', *, *, #15305, .F. ) ;
#35718=VECTOR ( 'NONE', #2490, 1000.000000000000114 ) ;
#35724=LINE ( 'NONE', #35950, #25017 ) ;
#35740=CIRCLE ( 'NONE', #40120, 5.500000000000001776 ) ;
#35743=AXIS2_PLACEMENT_3D ( 'NONE', #22345, #39219, #915 ) ;
#35752=CARTESIAN_POINT ( 'NONE',  ( -1.932019669644797988, -4.762702382056356321, -19.39321520033831447 ) ) ;
#35758=DIRECTION ( 'NONE',  ( -0.9908103287288504424, 0.1352586133457950590, -4.625929269271490844E-15 ) ) ;
#35760=CARTESIAN_POINT ( 'NONE',  ( -13.38024818871938670, -5.026574971259677227, -18.19321520033831874 ) ) ;
#35761=CARTESIAN_POINT ( 'NONE',  ( 61.87547515407200649, -14.47097414721605446, -17.80504224133693114 ) ) ;
#35771=CARTESIAN_POINT ( 'NONE',  ( 75.95778847736514194, -3.256761025687008537, -19.39321520033831447 ) ) ;
#35772=DIRECTION ( 'NONE',  ( -0.9908103287288504424, 0.1352586133457950590, 0.000000000000000000 ) ) ;
#35773=( LENGTH_UNIT ( ) NAMED_UNIT ( * ) SI_UNIT ( .MILLI., .METRE. ) );
#35785=EDGE_LOOP ( 'NONE', ( #27454, #11287, #14153, #29647 ) ) ;
#35809=DIRECTION ( 'NONE',  ( -0.7962509850245486076, -0.6049664196031347974, 0.000000000000000000 ) ) ;
#35821=DIRECTION ( 'NONE',  ( 0.000000000000000000, 0.000000000000000000, 1.000000000000000000 ) ) ;
#35843=EDGE_LOOP ( 'NONE', ( #2803, #21237 ) ) ;
#35852=CARTESIAN_POINT ( 'NONE',  ( 71.31713442278437753, 2.423123680056944007, -15.89321520033831447 ) ) ;
#35853=CIRCLE ( 'NONE', #42463, 5.500000000000001776 ) ;
#35863=PRODUCT_DEFINITION_FORMATION_WITH_SPECIFIED_SOURCE ( 'ANY', '', #35013, .NOT_KNOWN. ) ;
#35865=DIRECTION ( 'NONE',  ( 0.000000000000000000, 0.000000000000000000, -1.000000000000000000 ) ) ;
#35867=ADVANCED_FACE ( 'NONE', ( #40706 ), #23377, .T. ) ;
#35882=ADVANCED_FACE ( 'NONE', ( #9695 ), #20735, .T. ) ;
#35884=FACE_OUTER_BOUND ( 'NONE', #36712, .T. ) ;
#35887=VERTEX_POINT ( 'NONE', #16312 ) ;
#35898=CARTESIAN_POINT ( 'NONE',  ( 62.36331481590491421, -14.51968798477309797, -9.194700042550184804 ) ) ;
#35912=CARTESIAN_POINT ( 'NONE',  ( 64.65536759514621679, -15.48292270431935336, -11.12858986817582441 ) ) ;
#35940=CARTESIAN_POINT ( 'NONE',  ( 75.95778847736514194, -3.256761025687008537, -10.39321520033831625 ) ) ;
#35950=CARTESIAN_POINT ( 'NONE',  ( 77.44400397045842510, -3.459648945705700473, -7.147228641687434880 ) ) ;
#35960=CARTESIAN_POINT ( 'NONE',  ( 66.31316073997737703, -0.09061936939670083013, -16.39321520033831447 ) ) ;
#35987=ORIENTED_EDGE ( 'NONE', *, *, #40636, .F. ) ;
#35992=PRESENTATION_STYLE_ASSIGNMENT (( #39881 ) ) ;
#36027=ORIENTED_EDGE ( 'NONE', *, *, #27184, .T. ) ;
#36040=CARTESIAN_POINT ( 'NONE',  ( -13.49987324484352769, -3.923910153600668860, -18.82182469926544854 ) ) ;
#36059=FACE_OUTER_BOUND ( 'NONE', #9967, .T. ) ;
#36079=CYLINDRICAL_SURFACE ( 'NONE', #35655, 2.999999999999996003 ) ;
#36088=ORIENTED_EDGE ( 'NONE', *, *, #20436, .T. ) ;
#36101=CIRCLE ( 'NONE', #16466, 35.00000000000000000 ) ;
#36105=CARTESIAN_POINT ( 'NONE',  ( 0.04488520489200759078, -6.166763362545027327, -19.39321520033831447 ) ) ;
#36119=CARTESIAN_POINT ( 'NONE',  ( 63.28220228971554207, -14.74607418325012098, -9.753631345296810196 ) ) ;
#36127=CARTESIAN_POINT ( 'NONE',  ( 64.28447634061448923, -12.99130359988381755, -15.72333420167097096 ) ) ;
#36133=AXIS2_PLACEMENT_3D ( 'NONE', #21792, #10643, #6995 ) ;
#36134=DIRECTION ( 'NONE',  ( -0.1352586133457952255, -0.9908103287288504424, 0.000000000000000000 ) ) ;
#36135=CARTESIAN_POINT ( 'NONE',  ( 66.40653143407884329, -14.77812736305742547, -10.49134286602717658 ) ) ;
#36151=CARTESIAN_POINT ( 'NONE',  ( -13.52873657336266078, -4.831135987035605872, -8.722383338069434444 ) ) ;
#36155=FACE_OUTER_BOUND ( 'NONE', #26931, .T. ) ;
#36160=EDGE_CURVE ( 'NONE', #26749, #873, #39643, .T. ) ;
#36167=VECTOR ( 'NONE', #13914, 1000.000000000000000 ) ;
#36183=CARTESIAN_POINT ( 'NONE',  ( -13.82468485392153568, -4.441611705562402257, -8.282184520274741502 ) ) ;
#36192=EDGE_CURVE ( 'NONE', #5874, #11018, #84, .T. ) ;
#36194=AXIS2_PLACEMENT_3D ( 'NONE', #14775, #18646, #42820 ) ;
#36202=EDGE_LOOP ( 'NONE', ( #29475, #17238, #6667, #8040 ) ) ;
#36224=EDGE_CURVE ( 'NONE', #16401, #33252, #23303, .T. ) ;
#36238=CARTESIAN_POINT ( 'NONE',  ( 59.77100663911058120, -14.81899367705580595, -8.593215200338313764 ) ) ;
#36254=DIRECTION ( 'NONE',  ( 0.000000000000000000, 0.000000000000000000, -1.000000000000000000 ) ) ;
#36264=CARTESIAN_POINT ( 'NONE',  ( 75.63675420052337017, -42.57465691284114939, -15.89321520033831447 ) ) ;
#36290=ORIENTED_EDGE ( 'NONE', *, *, #39491, .F. ) ;
#36316=CARTESIAN_POINT ( 'NONE',  ( 66.02672340405024443, -2.161076072907569756, -17.98865292984563169 ) ) ;
#36330=ORIENTED_EDGE ( 'NONE', *, *, #13189, .T. ) ;
#36350=CARTESIAN_POINT ( 'NONE',  ( 65.37189491326753910, -13.54774410707433141, -14.64331257007126297 ) ) ;
#36357=CARTESIAN_POINT ( 'NONE',  ( -1.894019060673375332, -6.852671617155902339, -18.74982798469211787 ) ) ;
#36358=CARTESIAN_POINT ( 'NONE',  ( 64.78880510502027334, -15.59149258467484422, -11.31956754614451199 ) ) ;
#36363=DIRECTION ( 'NONE',  ( 0.000000000000000000, 0.000000000000000000, 1.000000000000000000 ) ) ;
#36366=B_SPLINE_CURVE_WITH_KNOTS ( 'NONE', 3,
 ( #30402, #43861, #40441, #19679, #26760, #19916, #33339, #2573, #2344, #5538, #39979, #9202, #1667, #19456, #5320, #40669, #36768, #30177, #32891, #22650, #36989, #33801, #23112, #12634, #8742, #44095, #44324, #25849 ),
 .UNSPECIFIED., .F., .F.,
 ( 4, 2, 2, 2, 1, 1, 2, 2, 2, 2, 1, 1, 2, 2, 2, 4 ),
 ( 0.000000000000000000, 0.1249999999999990563, 0.1874999999999982514, 0.2187499999999976685, 0.2343749999999973077, 0.2421874999999971412, 0.2460937499999970579, 0.2499999999999969746, 0.3749999999999961697, 0.4374999999999955036, 0.4687499999999955036, 0.4843749999999956146, 0.4921874999999955591, 0.4999999999999955036, 0.7499999999999976685, 1.000000000000000000 ),
 .UNSPECIFIED. ) ;
#36376=CARTESIAN_POINT ( 'NONE',  ( -13.67812064622776802, -4.634518106585512776, -18.88472069773969153 ) ) ;
#36383=VERTEX_POINT ( 'NONE', #43834 ) ;
#36401=CARTESIAN_POINT ( 'NONE',  ( -13.48327269170832565, -4.890975110956025773, -7.580226695745068355 ) ) ;
#36428=CIRCLE ( 'NONE', #28445, 4.499999999999996447 ) ;
#36450=AXIS2_PLACEMENT_3D ( 'NONE', #37688, #20149, #31065 ) ;
#36461=CARTESIAN_POINT ( 'NONE',  ( 59.62174278132244609, -14.86814543204979344, -8.593215200338315540 ) ) ;
#36466=ADVANCED_FACE ( 'NONE', ( #37658 ), #9859, .F. ) ;
#36467=EDGE_CURVE ( 'NONE', #166, #10084, #23991, .T. ) ;
#36470=DIRECTION ( 'NONE',  ( 0.000000000000000000, 0.000000000000000000, 1.000000000000000000 ) ) ;
#36476=CARTESIAN_POINT ( 'NONE',  ( 65.04064389207671582, -15.49774878834461056, -16.33482031564782488 ) ) ;
#36501=CARTESIAN_POINT ( 'NONE',  ( 59.24641515291911986, -13.72835195454734247, -18.19321520033831519 ) ) ;
#36504=ORIENTED_EDGE ( 'NONE', *, *, #26777, .T. ) ;
#36527=ADVANCED_FACE ( 'NONE', ( #6197, #34003 ), #34443, .T. ) ;
#36534=CARTESIAN_POINT ( 'NONE',  ( 80.41643495664496299, -3.865424785743087899, -16.39321520033831447 ) ) ;
#36544=CYLINDRICAL_SURFACE ( 'NONE', #36613, 8.000000000000000000 ) ;
#36552=DIRECTION ( 'NONE',  ( 0.000000000000000000, 0.000000000000000000, 1.000000000000000000 ) ) ;
#36573=ADVANCED_FACE ( 'NONE', ( #30819 ), #18253, .T. ) ;
#36574=DIRECTION ( 'NONE',  ( 0.000000000000000000, 0.000000000000000000, -1.000000000000000000 ) ) ;
#36578=CARTESIAN_POINT ( 'NONE',  ( 64.33685879144834985, -13.01308064423183986, -15.68040082802806978 ) ) ;
#36585=CARTESIAN_POINT ( 'NONE',  ( 67.31358133957452594, -0.1451868489720468947, -10.39321520033831625 ) ) ;
#36586=CARTESIAN_POINT ( 'NONE',  ( -2.478595920918978290, -7.028301761946200266, -19.25792888057430829 ) ) ;
#36590=ORIENTED_EDGE ( 'NONE', *, *, #14241, .T. ) ;
#36599=CARTESIAN_POINT ( 'NONE',  ( 9.052690036452151645, -4.182915634381243919, -8.893215200338314474 ) ) ;
#36610=VERTEX_POINT ( 'NONE', #28525 ) ;
#36613=AXIS2_PLACEMENT_3D ( 'NONE', #5318, #8297, #8973 ) ;
#36631=CARTESIAN_POINT ( 'NONE',  ( 68.14538754644013352, -1.022943911447667720, -16.39321520033830737 ) ) ;
#36635=( GEOMETRIC_REPRESENTATION_CONTEXT ( 3 ) GLOBAL_UNCERTAINTY_ASSIGNED_CONTEXT ( ( #28224 ) ) GLOBAL_UNIT_ASSIGNED_CONTEXT ( ( #35773, #42860, #8423 ) ) REPRESENTATION_CONTEXT ( 'NONE', 'WORKASPACE' ) );
#36686=LINE ( 'NONE', #26452, #35718 ) ;
#36694=CIRCLE ( 'NONE', #33812, 11.00000000000000000 ) ;
#36704=ORIENTED_EDGE ( 'NONE', *, *, #32690, .T. ) ;
#36712=EDGE_LOOP ( 'NONE', ( #30943, #22938, #42052, #5154, #11249 ) ) ;
#36740=CARTESIAN_POINT ( 'NONE',  ( 31.16856251326850824, -20.50830283073288385, -18.19321520033831519 ) ) ;
#36767=ORIENTED_EDGE ( 'NONE', *, *, #32690, .F. ) ;
#36768=CARTESIAN_POINT ( 'NONE',  ( -2.175944109879409449, -6.937465585941038348, -7.722225285168071274 ) ) ;
#36806=CARTESIAN_POINT ( 'NONE',  ( 67.17917282099325860, -0.1070896992261115427, -10.39321520033831447 ) ) ;
#36812=DIRECTION ( 'NONE',  ( 0.9908103287288505534, -0.1352586133457945317, 0.000000000000000000 ) ) ;
#36824=CARTESIAN_POINT ( 'NONE',  ( -13.50689678881128231, -4.859881301483246041, -18.09470388050485568 ) ) ;
#36853=CARTESIAN_POINT ( 'NONE',  ( 67.05222635936684128, -0.08653180621725030386, -16.39321520033831092 ) ) ;
#36872=DIRECTION ( 'NONE',  ( -0.1352586133458019424, -0.9908103287288495542, 0.000000000000000000 ) ) ;
#36898=ORIENTED_EDGE ( 'NONE', *, *, #20016, .F. ) ;
#36902=ORIENTED_EDGE ( 'NONE', *, *, #43987, .F. ) ;
#36909=VECTOR ( 'NONE', #23654, 1000.000000000000000 ) ;
#36955=VERTEX_POINT ( 'NONE', #12542 ) ;
#36963=AXIS2_PLACEMENT_3D ( 'NONE', #26118, #16547, #36812 ) ;
#36974=DIRECTION ( 'NONE',  ( 0.1352586133457950590, 0.9908103287288504424, 0.000000000000000000 ) ) ;
#36982=CARTESIAN_POINT ( 'NONE',  ( 42.36021970110777346, -12.73296999994090761, -7.393215200338315363 ) ) ;
#36989=CARTESIAN_POINT ( 'NONE',  ( -2.071618846624489585, -6.906063984103743891, -7.819288697422720702 ) ) ;
#37020=CARTESIAN_POINT ( 'NONE',  ( 60.45894907855897316, -4.846173528048923096, -17.39321520033831447 ) ) ;
#37031=CARTESIAN_POINT ( 'NONE',  ( 3.060777270043529619, -5.064559853354640317, -19.39321520033831447 ) ) ;
#37032=CARTESIAN_POINT ( 'NONE',  ( -3.075987277002700804, -7.207016596002322473, -19.39321520033831447 ) ) ;
#37048=CARTESIAN_POINT ( 'NONE',  ( -13.73291115513471716, -3.820450301670890614, -18.35493171628743170 ) ) ;
#37080=CARTESIAN_POINT ( 'NONE',  ( 9.052690036452151645, -4.182915634381243919, -19.39321520033831447 ) ) ;
#37084=ORIENTED_EDGE ( 'NONE', *, *, #39891, .F. ) ;
#37107=CARTESIAN_POINT ( 'NONE',  ( 59.75121349346655109, -13.58877957849837692, -19.38162691376808411 ) ) ;
#37111=AXIS2_PLACEMENT_3D ( 'NONE', #31027, #38091, #17140 ) ;
#37121=ORIENTED_EDGE ( 'NONE', *, *, #6437, .T. ) ;
#37148=CARTESIAN_POINT ( 'NONE',  ( 27.78057335388972504, -13.48551096636548330, -17.89321520033831447 ) ) ;
#37152=ORIENTED_EDGE ( 'NONE', *, *, #22385, .F. ) ;
#37154=LINE ( 'NONE', #6618, #39440 ) ;
#37164=VECTOR ( 'NONE', #42123, 1000.000000000000000 ) ;
#37186=CARTESIAN_POINT ( 'NONE',  ( -7.917624645353497748, -12.21642755857638818, -19.39321520033831447 ) ) ;
#37187=EDGE_LOOP ( 'NONE', ( #22631, #5717, #22558, #13373 ) ) ;
#37196=CARTESIAN_POINT ( 'NONE',  ( 63.74703025577719018, -40.95155355269160680, -19.39321520033831447 ) ) ;
#37200=CARTESIAN_POINT ( 'NONE',  ( 59.44377208703740223, -12.82110557137145967, -17.39288367676203606 ) ) ;
#37214=CARTESIAN_POINT ( 'NONE',  ( 64.63131511434168885, -2.693399871814762925, -18.62537188001541466 ) ) ;
#37236=ADVANCED_FACE ( 'NONE', ( #44913 ), #17316, .T. ) ;
#37251=ORIENTED_EDGE ( 'NONE', *, *, #26503, .T. ) ;
#37255=EDGE_CURVE ( 'NONE', #2056, #36383, #2714, .T. ) ;
#37256=CARTESIAN_POINT ( 'NONE',  ( 66.84025912450881890, -0.06488636359980230750, -10.39321520033831625 ) ) ;
#37263=EDGE_LOOP ( 'NONE', ( #43225, #25377, #15125, #42641 ) ) ;
#37266=B_SPLINE_CURVE_WITH_KNOTS ( 'NONE', 3,
 ( #35129, #28995, #32175, #8241, #10995, #36040, #11221, #31947, #18730, #25127 ),
 .UNSPECIFIED., .F., .F.,
 ( 4, 2, 2, 2, 4 ),
 ( 5.485677294651094893E-18, 0.0005882757591493389601, 0.001176551518298672282, 0.001764827277448005821, 0.002353103036597339361 ),
 .UNSPECIFIED. ) ;
#37286=EDGE_LOOP ( 'NONE', ( #27028, #38472, #28108, #2755, #39040, #7922, #13734, #2271, #21612, #36088 ) ) ;
#37293=ORIENTED_EDGE ( 'NONE', *, *, #25630, .F. ) ;
#37312=CARTESIAN_POINT ( 'NONE',  ( 65.55689610126231059, -13.67296395165911704, -14.39321520033831625 ) ) ;
#37329=ADVANCED_FACE ( 'NONE', ( #20952 ), #10473, .T. ) ;
#37351=PLANE ( 'NONE',  #11140 ) ;
#37369=CARTESIAN_POINT ( 'NONE',  ( -7.923679509334008664, -5.078949698970065540, -19.39321520033831447 ) ) ;
#37375=AXIS2_PLACEMENT_3D ( 'NONE', #14318, #20502, #17084 ) ;
#37427=CARTESIAN_POINT ( 'NONE',  ( 31.16856251326850824, -20.50830283073288385, -19.39321520033831447 ) ) ;
#37454=DIRECTION ( 'NONE',  ( 0.9908103287288502203, -0.1352586133457981954, 0.000000000000000000 ) ) ;
#37505=DIRECTION ( 'NONE',  ( -0.9908103287288504424, 0.1352586133457950313, 0.000000000000000000 ) ) ;
#37546=AXIS2_PLACEMENT_3D ( 'NONE', #8446, #33485, #2263 ) ;
#37549=B_SPLINE_CURVE_WITH_KNOTS ( 'NONE', 3,
 ( #7854, #25186, #11279, #21310, #18342, #39312, #35421, #3969, #32008, #31788, #560, #21533, #35652, #28378, #42291, #24956, #38852, #18115, #772, #14695, #39085, #21760, #4426, #32235, #6867, #37649, #44958, #17359, #23759, #24415, #10514, #44502, #10079, #6646, #20554, #2990, #16916, #13715, #7083, #27171, #34435 ),
 .UNSPECIFIED., .F., .F.,
 ( 4, 2, 1, 1, 1, 2, 2, 2, 1, 1, 1, 2, 2, 2, 2, 1, 1, 2, 2, 2, 2, 1, 2, 2, 4 ),
 ( 0.000000000000000000, 0.06249999999992449096, 0.09374999999988881116, 0.1093749999998711170, 0.1171874999998622630, 0.1210937499998595568, 0.1249999999998568645, 0.1874999999998673561, 0.2187499999998746836, 0.2343749999998763767, 0.2421874999998769873, 0.2460937499998774036, 0.2499999999998778200, 0.3749999999999229505, 0.4374999999999431011, 0.4687499999999530931, 0.4843749999999580891, 0.4921874999999604761, 0.4999999999999629186, 0.6249999999999770184, 0.6874999999999841238, 0.7187499999999891198, 0.7343749999999902300, 0.7499999999999912292, 1.000000000000000000 ),
 .UNSPECIFIED. ) ;
#37551=LINE ( 'NONE', #20241, #25534 ) ;
#37553=ORIENTED_EDGE ( 'NONE', *, *, #38102, .T. ) ;
#37558=EDGE_CURVE ( 'NONE', #854, #26347, #133, .T. ) ;
#37567=CIRCLE ( 'NONE', #44878, 26.50000000000000000 ) ;
#37583=AXIS2_PLACEMENT_3D ( 'NONE', #21480, #35365, #32180 ) ;
#37592=ORIENTED_EDGE ( 'NONE', *, *, #6114, .T. ) ;
#37616=VERTEX_POINT ( 'NONE', #2200 ) ;
#37628=DIRECTION ( 'NONE',  ( -0.9908103287288505534, 0.1352586133457950590, 0.000000000000000000 ) ) ;
#37649=CARTESIAN_POINT ( 'NONE',  ( 63.02684575864485339, -12.60992855379462618, -10.24602201293989978 ) ) ;
#37658=FACE_OUTER_BOUND ( 'NONE', #12419, .T. ) ;
#37660=TOROIDAL_SURFACE ( 'NONE', #1261, 8.800000000000000711, 1.199999999999999956 ) ;
#37688=CARTESIAN_POINT ( 'NONE',  ( 31.33087284928348026, -19.31933043625826585, -8.593215200338315540 ) ) ;
#37762=CARTESIAN_POINT ( 'NONE',  ( 42.57150613532612482, -13.18613447638990088, -14.39321520033831625 ) ) ;
#37765=CARTESIAN_POINT ( 'NONE',  ( 61.14763380861215580, -2.318372254017448508, -8.893215200339504634 ) ) ;
#37812=EDGE_CURVE ( 'NONE', #6454, #6765, #35272, .T. ) ;
#37819=DIRECTION ( 'NONE',  ( 0.000000000000000000, 0.000000000000000000, -1.000000000000000000 ) ) ;
#37845=DIRECTION ( 'NONE',  ( 0.000000000000000000, 0.000000000000000000, -1.000000000000000000 ) ) ;
#37847=EDGE_CURVE ( 'NONE', #18952, #2128, #38254, .T. ) ;
#37850=EDGE_LOOP ( 'NONE', ( #3760, #5311, #39822, #38865 ) ) ;
#37857=DIRECTION ( 'NONE',  ( -0.9908103287288501093, 0.1352586133457976958, 0.000000000000000000 ) ) ;
#37866=ADVANCED_FACE ( 'NONE', ( #7414 ), #3554, .F. ) ;
#37899=EDGE_LOOP ( 'NONE', ( #32411, #2083, #24175, #38170 ) ) ;
#37902=CARTESIAN_POINT ( 'NONE',  ( 59.24641515291911986, -13.72835195454734425, -19.39321520033831803 ) ) ;
#37922=ADVANCED_FACE ( 'NONE', ( #26101 ), #8552, .F. ) ;
#37929=VERTEX_POINT ( 'NONE', #21786 ) ;
#37939=CARTESIAN_POINT ( 'NONE',  ( 62.66445125428926843, -3.444971829879546643, -7.594369504596270026 ) ) ;
#37961=DIRECTION ( 'NONE',  ( -1.000000000000000000, 0.000000000000000000, 0.000000000000000000 ) ) ;
#37965=AXIS2_PLACEMENT_3D ( 'NONE', #1397, #25362, #29442 ) ;
#38000=CARTESIAN_POINT ( 'NONE',  ( 35.67453213195965134, -67.60842401891365228, -7.393215200338315363 ) ) ;
#38035=CIRCLE ( 'NONE', #39503, 33.80000000000000426 ) ;
#38036=EDGE_CURVE ( 'NONE', #40192, #26749, #18373, .T. ) ;
#38039=ORIENTED_EDGE ( 'NONE', *, *, #276, .F. ) ;
#38068=DIRECTION ( 'NONE',  ( 0.000000000000000000, 0.000000000000000000, 1.000000000000000000 ) ) ;
#38083=ORIENTED_EDGE ( 'NONE', *, *, #23688, .F. ) ;
#38086=CIRCLE ( 'NONE', #33711, 33.80000000000000426 ) ;
#38089=ORIENTED_EDGE ( 'NONE', *, *, #36192, .F. ) ;
#38091=DIRECTION ( 'NONE',  ( 0.4225728684367167087, -0.9063289528979890930, -0.000000000000000000 ) ) ;
#38102=EDGE_CURVE ( 'NONE', #38550, #13151, #41707, .T. ) ;
#38108=DIRECTION ( 'NONE',  ( 0.9908103287288504424, -0.1352586133457952533, 0.000000000000000000 ) ) ;
#38128=DIRECTION ( 'NONE',  ( -0.1352586133457951423, -0.9908103287288504424, 0.000000000000000000 ) ) ;
#38149=ADVANCED_FACE ( 'NONE', ( #20570 ), #13279, .T. ) ;
#38155=ORIENTED_EDGE ( 'NONE', *, *, #18920, .F. ) ;
#38156=CARTESIAN_POINT ( 'NONE',  ( 59.58307739690713589, -13.63526775528383794, -7.397079453926873605 ) ) ;
#38170=ORIENTED_EDGE ( 'NONE', *, *, #276, .T. ) ;
#38181=DIRECTION ( 'NONE',  ( -1.000000000000000000, 0.000000000000000000, 0.000000000000000000 ) ) ;
#38187=LINE ( 'NONE', #44828, #13107 ) ;
#38200=VECTOR ( 'NONE', #7415, 1000.000000000000000 ) ;
#38229=EDGE_CURVE ( 'NONE', #1626, #259, #19326, .T. ) ;
#38233=ADVANCED_FACE ( 'NONE', ( #41551 ), #22253, .T. ) ;
#38237=DIRECTION ( 'NONE',  ( 0.9908103287288504424, -0.1352586133457950035, 0.000000000000000000 ) ) ;
#38238=VERTEX_POINT ( 'NONE', #6879 ) ;
#38254=CIRCLE ( 'NONE', #10620, 0.5000000000000004441 ) ;
#38260=DIRECTION ( 'NONE',  ( 0.9908103287288504424, -0.1352586133457950590, 0.000000000000000000 ) ) ;
#38280=VERTEX_POINT ( 'NONE', #1370 ) ;
#38315=CARTESIAN_POINT ( 'NONE',  ( 80.91184012100937650, -3.933054092416038650, -15.89321520033831447 ) ) ;
#38334=ORIENTED_EDGE ( 'NONE', *, *, #38394, .T. ) ;
#38340=CARTESIAN_POINT ( 'NONE',  ( -1.145390592550938891, -14.88589425535892019, -18.19321520033831519 ) ) ;
#38355=AXIS2_PLACEMENT_3D ( 'NONE', #22928, #1722, #12455 ) ;
#38369=EDGE_LOOP ( 'NONE', ( #42012, #36027, #33999, #13497 ) ) ;
#38394=EDGE_CURVE ( 'NONE', #41326, #12923, #11323, .T. ) ;
#38417=ADVANCED_FACE ( 'NONE', ( #7990 ), #32378, .T. ) ;
#38457=DIRECTION ( 'NONE',  ( 0.000000000000000000, 0.000000000000000000, 1.000000000000000000 ) ) ;
#38472=ORIENTED_EDGE ( 'NONE', *, *, #7095, .T. ) ;
#38500=CARTESIAN_POINT ( 'NONE',  ( 61.15357748477988764, -14.46166092335914755, -19.21272425282928964 ) ) ;
#38511=DIRECTION ( 'NONE',  ( 0.1352586133457905626, 0.9908103287288509975, 0.000000000000000000 ) ) ;
#38532=CARTESIAN_POINT ( 'NONE',  ( 59.39246203831174853, -12.83800168394059682, -9.393215200338312698 ) ) ;
#38535=DIRECTION ( 'NONE',  ( -0.9908103287288504424, 0.1352586133457954476, 0.000000000000000000 ) ) ;
#38547=ADVANCED_FACE ( 'NONE', ( #28976 ), #35336, .F. ) ;
#38550=VERTEX_POINT ( 'NONE', #31703 ) ;
#38560=ORIENTED_EDGE ( 'NONE', *, *, #21494, .F. ) ;
#38609=CARTESIAN_POINT ( 'NONE',  ( 61.55121550909755257, -14.46605081255149905, -17.91752732931888303 ) ) ;
#38636=AXIS2_PLACEMENT_3D ( 'NONE', #25349, #39243, #35809 ) ;
#38650=EDGE_CURVE ( 'NONE', #19947, #42200, #12076, .T. ) ;
#38652=CARTESIAN_POINT ( 'NONE',  ( 75.14134903615895666, -42.50702760616825771, -16.39321520033831447 ) ) ;
#38653=DIRECTION ( 'NONE',  ( 0.000000000000000000, 0.000000000000000000, 1.000000000000000000 ) ) ;
#38702=FACE_OUTER_BOUND ( 'NONE', #40348, .T. ) ;
#38728=CARTESIAN_POINT ( 'NONE',  ( 65.34856691214200453, -14.13229026159626045, -17.32302191349986487 ) ) ;
#38762=CARTESIAN_POINT ( 'NONE',  ( 60.06931813437629586, -14.72076136720887085, -18.18301750815651374 ) ) ;
#38777=DIRECTION ( 'NONE',  ( 0.000000000000000000, 0.000000000000000000, -1.000000000000000000 ) ) ;
#38804=EDGE_LOOP ( 'NONE', ( #38039, #37293 ) ) ;
#38811=DIRECTION ( 'NONE',  ( -0.9908103287288504424, 0.1352586133457950035, 0.000000000000000000 ) ) ;
#38852=CARTESIAN_POINT ( 'NONE',  ( 64.41506894153299356, -13.04641652406104946, -11.17147419670170194 ) ) ;
#38865=ORIENTED_EDGE ( 'NONE', *, *, #31425, .T. ) ;
#38871=CARTESIAN_POINT ( 'NONE',  ( 60.91427317013854292, -14.50360402731886644, -8.693199542283664982 ) ) ;
#38878=DIRECTION ( 'NONE',  ( -1.000000000000000000, 0.000000000000000000, 0.000000000000000000 ) ) ;
#38884=CARTESIAN_POINT ( 'NONE',  ( 64.81496985121363252, -15.50732193479129606, -9.201218580878807174 ) ) ;
#38909=CARTESIAN_POINT ( 'NONE',  ( 63.56235174433628998, -1.192518024930046661, -17.37770299495512205 ) ) ;
#38928=CARTESIAN_POINT ( 'NONE',  ( 64.67456875498254476, -2.676871470862063340, -8.178078223173255168 ) ) ;
#38929=FACE_OUTER_BOUND ( 'NONE', #21323, .T. ) ;
#38940=VECTOR ( 'NONE', #37819, 1000.000000000000000 ) ;
#38959=CARTESIAN_POINT ( 'NONE',  ( -13.32377113153209791, -5.100909530930220370, -18.19321520033831874 ) ) ;
#38960=CARTESIAN_POINT ( 'NONE',  ( 64.81488287508310009, -15.50725790103587087, -17.58527714782560025 ) ) ;
#38978=AXIS2_PLACEMENT_3D ( 'NONE', #43212, #40238, #22007 ) ;
#38992=DIRECTION ( 'NONE',  ( -0.3127730236694426513, 0.9498278979187093629, 0.000000000000000000 ) ) ;
#39021=CARTESIAN_POINT ( 'NONE',  ( 65.48165112743716065, -14.20078584921842513, -17.21198551020792067 ) ) ;
#39040=ORIENTED_EDGE ( 'NONE', *, *, #42868, .T. ) ;
#39048=VERTEX_POINT ( 'NONE', #1317 ) ;
#39063=FACE_OUTER_BOUND ( 'NONE', #36202, .T. ) ;
#39079=CYLINDRICAL_SURFACE ( 'NONE', #24108, 0.5000000000000039968 ) ;
#39085=CARTESIAN_POINT ( 'NONE',  ( 63.90740853991285064, -12.84492318790033138, -10.77114471798664042 ) ) ;
#39098=ORIENTED_EDGE ( 'NONE', *, *, #18106, .T. ) ;
#39119=CARTESIAN_POINT ( 'NONE',  ( 65.58071483341541352, -14.25348465845825707, -9.659601953590369661 ) ) ;
#39123=ORIENTED_EDGE ( 'NONE', *, *, #13627, .F. ) ;
#39124=DIRECTION ( 'NONE',  ( 0.1352586133457950590, 0.9908103287288504424, 0.000000000000000000 ) ) ;
#39162=CARTESIAN_POINT ( 'NONE',  ( -13.73225313964263172, -3.820740757134447829, -8.430338879382498263 ) ) ;
#39188=CARTESIAN_POINT ( 'NONE',  ( 59.58306117764126952, -13.63527223977064118, -19.38935169184939156 ) ) ;
#39197=VECTOR ( 'NONE', #215, 1000.000000000000000 ) ;
#39219=DIRECTION ( 'NONE',  ( 0.000000000000000000, 0.000000000000000000, 1.000000000000000000 ) ) ;
#39232=ADVANCED_FACE ( 'NONE', ( #16823 ), #34124, .T. ) ;
#39243=DIRECTION ( 'NONE',  ( -0.6049664196031347974, 0.7962509850245486076, 0.000000000000000000 ) ) ;
#39264=ADVANCED_FACE ( 'NONE', ( #34345 ), #24109, .F. ) ;
#39266=AXIS2_PLACEMENT_3D ( 'NONE', #35940, #15658, #11789 ) ;
#39269=ORIENTED_EDGE ( 'NONE', *, *, #1035, .F. ) ;
#39289=EDGE_LOOP ( 'NONE', ( #25146, #22995, #2464, #22586 ) ) ;
#39305=CARTESIAN_POINT ( 'NONE',  ( 61.76166819790555707, -14.46743153019225048, -17.84642471321736679 ) ) ;
#39312=CARTESIAN_POINT ( 'NONE',  ( 65.09033057751396711, -13.38310350479848054, -11.82419014234386268 ) ) ;
#39324=CYLINDRICAL_SURFACE ( 'NONE', #23289, 9.999999999999998224 ) ;
#39339=AXIS2_PLACEMENT_3D ( 'NONE', #25331, #32377, #7309 ) ;
#39344=CARTESIAN_POINT ( 'NONE',  ( -13.78505786849281911, -3.796669023460694792, -8.893215200338314474 ) ) ;
#39349=CARTESIAN_POINT ( 'NONE',  ( 61.95514858534045288, -14.46403247248995427, -7.783443800098010179 ) ) ;
#39376=VERTEX_POINT ( 'NONE', #16593 ) ;
#39378=VECTOR ( 'NONE', #30458, 1000.000000000000000 ) ;
#39389=ORIENTED_EDGE ( 'NONE', *, *, #38650, .T. ) ;
#39394=CARTESIAN_POINT ( 'NONE',  ( -13.32377113153209791, -5.100909530930222147, -8.593215200338315540 ) ) ;
#39395=CIRCLE ( 'NONE', #76, 5.500000000000001776 ) ;
#39396=CARTESIAN_POINT ( 'NONE',  ( 64.24243542014160369, -41.01918285936451269, -10.39321520033831625 ) ) ;
#39398=CARTESIAN_POINT ( 'NONE',  ( 65.72288960572690542, -0.2187004563819841818, -16.39321520033831803 ) ) ;
#39418=CARTESIAN_POINT ( 'NONE',  ( 59.75121349346655109, -13.58877957849837692, -7.404803486908546617 ) ) ;
#39422=CARTESIAN_POINT ( 'NONE',  ( 62.22090115686911815, -14.48605130139344332, -18.92121278399942952 ) ) ;
#39440=VECTOR ( 'NONE', #9825, 1000.000000000000000 ) ;
#39442=DIRECTION ( 'NONE',  ( 0.000000000000000000, 0.000000000000000000, 1.000000000000000000 ) ) ;
#39449=VERTEX_POINT ( 'NONE', #38652 ) ;
#39456=CARTESIAN_POINT ( 'NONE',  ( -12.61278219666105649, -4.053125158562568942, -17.89321520033831447 ) ) ;
#39491=EDGE_CURVE ( 'NONE', #41326, #44000, #10678, .T. ) ;
#39503=AXIS2_PLACEMENT_3D ( 'NONE', #7757, #21665, #18246 ) ;
#39520=EDGE_LOOP ( 'NONE', ( #30111, #34489, #27481, #23228, #2048, #35210, #42354, #20037, #1173, #5880, #11597, #24826 ) ) ;
#39525=CARTESIAN_POINT ( 'NONE',  ( -1.637506834317598026, -6.775152287193681566, -17.89321520033831447 ) ) ;
#39574=CARTESIAN_POINT ( 'NONE',  ( -1.667125815598008209, -6.784308745172333843, -18.25434776483827193 ) ) ;
#39575=CARTESIAN_POINT ( 'NONE',  ( 63.19922959105626603, -13.42641530295352403, -8.168935231742574743 ) ) ;
#39595=CARTESIAN_POINT ( 'NONE',  ( -13.43397602290982462, -4.955858912465142652, -18.16431974193844923 ) ) ;
#39622=DIRECTION ( 'NONE',  ( -0.1352586133457952255, -0.9908103287288504424, 0.000000000000000000 ) ) ;
#39624=CARTESIAN_POINT ( 'NONE',  ( 67.12658297191856605, -0.09863003671598137567, -16.39321520033831447 ) ) ;
#39643=CIRCLE ( 'NONE', #44772, 5.000000000000000000 ) ;
#39649=CARTESIAN_POINT ( 'NONE',  ( -13.50731098778515538, -4.859336136776158277, -18.09677371840150784 ) ) ;
#39659=LINE ( 'NONE', #43531, #41711 ) ;
#39687=CARTESIAN_POINT ( 'NONE',  ( 65.41257106814472877, -15.47412461924279725, -16.39321520033831447 ) ) ;
#39715=VERTEX_POINT ( 'NONE', #24988 ) ;
#39720=CARTESIAN_POINT ( 'NONE',  ( 41.72636039845269096, -11.37347657059392070, -16.39321520033831447 ) ) ;
#39724=ORIENTED_EDGE ( 'NONE', *, *, #25630, .T. ) ;
#39773=VECTOR ( 'NONE', #21428, 1000.000000000000000 ) ;
#39782=LINE ( 'NONE', #40471, #14659 ) ;
#39786=CARTESIAN_POINT ( 'NONE',  ( 64.35925685210249014, -13.02253225675024240, -15.66181482168427586 ) ) ;
#39794=CARTESIAN_POINT ( 'NONE',  ( -2.049502439613130278, -6.899408072110920997, -18.94416755177243061 ) ) ;
#39795=CARTESIAN_POINT ( 'NONE',  ( 62.23965954364707898, -13.31694178448660004, -7.820742382077911614 ) ) ;
#39815=CARTESIAN_POINT ( 'NONE',  ( -13.75549929796900273, -4.532673069121776699, -18.69989194241940922 ) ) ;
#39822=ORIENTED_EDGE ( 'NONE', *, *, #42726, .F. ) ;
#39824=EDGE_CURVE ( 'NONE', #30249, #36383, #22915, .T. ) ;
#39853=AXIS2_PLACEMENT_3D ( 'NONE', #24259, #28568, #38811 ) ;
#39866=CARTESIAN_POINT ( 'NONE',  ( 46.47434218039879283, -17.93412427487546523, -18.19321520033831519 ) ) ;
#39881=SURFACE_STYLE_USAGE ( .BOTH. , #15038 ) ;
#39891=EDGE_CURVE ( 'NONE', #40192, #4744, #3828, .T. ) ;
#39921=ORIENTED_EDGE ( 'NONE', *, *, #14170, .F. ) ;
#39930=ORIENTED_EDGE ( 'NONE', *, *, #19476, .F. ) ;
#39940=ADVANCED_FACE ( 'NONE', ( #6497, #23150, #6268 ), #12899, .F. ) ;
#39949=VERTEX_POINT ( 'NONE', #23840 ) ;
#39979=CARTESIAN_POINT ( 'NONE',  ( -2.543030055175557802, -7.047612661366984277, -7.499921549712347257 ) ) ;
#40017=CARTESIAN_POINT ( 'NONE',  ( 65.88020736227775842, -0.1838173346746251047, -10.39321520033831625 ) ) ;
#40018=CARTESIAN_POINT ( 'NONE',  ( -2.398579840503125560, -7.004315730407527418, -19.21681588960016640 ) ) ;
#40019=CARTESIAN_POINT ( 'NONE',  ( 66.31928500851137187, -14.71576354012722021, -10.39321520033831625 ) ) ;
#40065=CARTESIAN_POINT ( 'NONE',  ( 67.01977926936005758, -0.08205263468559398365, -16.39321520033831092 ) ) ;
#40120=AXIS2_PLACEMENT_3D ( 'NONE', #11957, #32462, #11729 ) ;
#40122=CARTESIAN_POINT ( 'NONE',  ( 59.92022724782403742, -14.76985616374063248, -8.596615087808567424 ) ) ;
#40124=AXIS2_PLACEMENT_3D ( 'NONE', #26239, #13416, #20479 ) ;
#40126=EDGE_CURVE ( 'NONE', #11850, #42225, #1283, .T. ) ;
#40170=ORIENTED_EDGE ( 'NONE', *, *, #28069, .T. ) ;
#40192=VERTEX_POINT ( 'NONE', #39525 ) ;
#40194=CYLINDRICAL_SURFACE ( 'NONE', #19115, 0.5000000000000039968 ) ;
#40206=PLANE ( 'NONE',  #41078 ) ;
#40217=CYLINDRICAL_SURFACE ( 'NONE', #25579, 10.00000000000000000 ) ;
#40237=CARTESIAN_POINT ( 'NONE',  ( 59.24641515291911986, -13.72835195454734425, -7.393215200338315363 ) ) ;
#40238=DIRECTION ( 'NONE',  ( 0.000000000000000000, 0.000000000000000000, -1.000000000000000000 ) ) ;
#40256=PLANE ( 'NONE',  #25865 ) ;
#40257=CARTESIAN_POINT ( 'NONE',  ( 66.27224413149734517, -14.92707987627686350, -10.39321520033831803 ) ) ;
#40291=ORIENTED_EDGE ( 'NONE', *, *, #36224, .T. ) ;
#40297=CARTESIAN_POINT ( 'NONE',  ( 67.57613997102261294, -0.2549909087870869118, -16.39321520033831447 ) ) ;
#40326=VERTEX_POINT ( 'NONE', #36534 ) ;
#40348=EDGE_LOOP ( 'NONE', ( #15109, #33240, #34015, #11650 ) ) ;
#40355=LINE ( 'NONE', #19832, #27012 ) ;
#40412=CARTESIAN_POINT ( 'NONE',  ( 65.41257106814472877, -15.47412461924279725, -16.39321520033831447 ) ) ;
#40422=ORIENTED_EDGE ( 'NONE', *, *, #9793, .F. ) ;
#40437=CARTESIAN_POINT ( 'NONE',  ( 62.61908855860606593, -3.462305083068016209, -19.20062954177708647 ) ) ;
#40441=CARTESIAN_POINT ( 'NONE',  ( -2.989272046485941914, -7.181056780202320411, -7.392714882508171215 ) ) ;
#40471=CARTESIAN_POINT ( 'NONE',  ( 59.36680634945872725, -12.84644995903807896, -19.39321520033831447 ) ) ;
#40475=ORIENTED_EDGE ( 'NONE', *, *, #31425, .F. ) ;
#40480=CARTESIAN_POINT ( 'NONE',  ( 67.63289214294319152, -0.2818690679646981834, -10.39321520033831625 ) ) ;
#40482=DIRECTION ( 'NONE',  ( -0.4225728684367169308, 0.9063289528979889820, 0.000000000000000000 ) ) ;
#40484=VECTOR ( 'NONE', #34526, 1000.000000000000000 ) ;
#40486=EDGE_LOOP ( 'NONE', ( #18664, #19651, #30565, #21933, #6852, #28766 ) ) ;
#40488=CARTESIAN_POINT ( 'NONE',  ( 65.62759297140451054, -15.45042670135892671, -10.39321520033831803 ) ) ;
#40530=CIRCLE ( 'NONE', #32472, 6.000000000000005329 ) ;
#40541=DIRECTION ( 'NONE',  ( 0.000000000000000000, 0.000000000000000000, -1.000000000000000000 ) ) ;
#40565=CARTESIAN_POINT ( 'NONE',  ( 67.08264006073221708, -20.21382323020432992, -16.39321520033831447 ) ) ;
#40579=DIRECTION ( 'NONE',  ( 0.000000000000000000, 0.000000000000000000, -1.000000000000000000 ) ) ;
#40631=ORIENTED_EDGE ( 'NONE', *, *, #42046, .F. ) ;
#40632=ORIENTED_EDGE ( 'NONE', *, *, #11962, .F. ) ;
#40636=EDGE_CURVE ( 'NONE', #39949, #18111, #11537, .T. ) ;
#40644=DIRECTION ( 'NONE',  ( 0.000000000000000000, 0.000000000000000000, 1.000000000000000000 ) ) ;
#40646=EDGE_LOOP ( 'NONE', ( #4434, #42637, #2343, #31490 ) ) ;
#40650=CARTESIAN_POINT ( 'NONE',  ( 72.51188087854242781, -21.10583385764521225, -17.89321520033831447 ) ) ;
#40657=EDGE_CURVE ( 'NONE', #18680, #20781, #10428, .T. ) ;
#40659=CARTESIAN_POINT ( 'NONE',  ( 59.58307739690713589, -13.63526775528386459, -19.38935094674975801 ) ) ;
#40669=CARTESIAN_POINT ( 'NONE',  ( -2.210854019365580569, -6.947965325911625634, -7.693738507800350845 ) ) ;
#40675=CARTESIAN_POINT ( 'NONE',  ( 64.73784058450603140, -41.08681216603740438, -10.39321520033831625 ) ) ;
#40692=DIRECTION ( 'NONE',  ( 0.1352586133457952255, 0.9908103287288504424, 0.000000000000000000 ) ) ;
#40694=EDGE_CURVE ( 'NONE', #2987, #31347, #4210, .T. ) ;
#40704=CARTESIAN_POINT ( 'NONE',  ( 66.43257361571872366, -0.06953383795915370202, -10.39321520033831447 ) ) ;
#40706=FACE_OUTER_BOUND ( 'NONE', #1611, .T. ) ;
#40713=EDGE_CURVE ( 'NONE', #6765, #1626, #34785, .T. ) ;
#40716=FACE_OUTER_BOUND ( 'NONE', #40646, .T. ) ;
#40827=ORIENTED_EDGE ( 'NONE', *, *, #9452, .F. ) ;
#40832=ADVANCED_FACE ( 'NONE', ( #35461 ), #4236, .F. ) ;
#40850=DIRECTION ( 'NONE',  ( 0.9063289528979890930, 0.4225728684367167087, 0.000000000000000000 ) ) ;
#40858=ORIENTED_EDGE ( 'NONE', *, *, #29281, .F. ) ;
#40865=ORIENTED_EDGE ( 'NONE', *, *, #41467, .T. ) ;
#40900=ORIENTED_EDGE ( 'NONE', *, *, #37558, .T. ) ;
#40925=ADVANCED_FACE ( 'NONE', ( #2615 ), #11520, .T. ) ;
#40928=FACE_OUTER_BOUND ( 'NONE', #5071, .T. ) ;
#40965=ORIENTED_EDGE ( 'NONE', *, *, #2147, .T. ) ;
#40972=ORIENTED_EDGE ( 'NONE', *, *, #13500, .F. ) ;
#40984=CARTESIAN_POINT ( 'NONE',  ( 61.35533094128319931, -2.221534154745201217, -7.278987677919483978 ) ) ;
#40996=CARTESIAN_POINT ( 'NONE',  ( -12.61278219666105826, -4.053125158562569830, -19.39321520033831447 ) ) ;
#41005=AXIS2_PLACEMENT_3D ( 'NONE', #15487, #12750, #15942 ) ;
#41075=ORIENTED_EDGE ( 'NONE', *, *, #4943, .F. ) ;
#41078=AXIS2_PLACEMENT_3D ( 'NONE', #22424, #19002, #8739 ) ;
#41099=ADVANCED_FACE ( 'NONE', ( #26800, #6035, #43672 ), #40256, .F. ) ;
#41105=CARTESIAN_POINT ( 'NONE',  ( 70.97035005826803911, 2.261436620216128013, -16.39321520033831447 ) ) ;
#41132=DIRECTION ( 'NONE',  ( 0.9063289528979890930, 0.4225728684367167087, 0.000000000000000000 ) ) ;
#41146=ORIENTED_EDGE ( 'NONE', *, *, #43987, .T. ) ;
#41166=DIRECTION ( 'NONE',  ( 0.000000000000000000, 0.000000000000000000, -1.000000000000000000 ) ) ;
#41192=ORIENTED_EDGE ( 'NONE', *, *, #10274, .F. ) ;
#41201=CIRCLE ( 'NONE', #8400, 1.200000000000000622 ) ;
#41206=EDGE_LOOP ( 'NONE', ( #29731, #29047, #6416, #41558, #41146, #36767, #8057, #10353 ) ) ;
#41207=CARTESIAN_POINT ( 'NONE',  ( 62.38867158002533841, -1.739742509014211791, -9.130636672632755690 ) ) ;
#41219=EDGE_CURVE ( 'NONE', #33252, #8541, #19965, .T. ) ;
#41225=DIRECTION ( 'NONE',  ( -0.1352586133457950590, -0.9908103287288504424, 0.000000000000000000 ) ) ;
#41244=CARTESIAN_POINT ( 'NONE',  ( 46.84966980880212617, -19.07391775237791620, -8.593215200338315540 ) ) ;
#41247=EDGE_CURVE ( 'NONE', #34939, #4744, #17891, .T. ) ;
#41263=ORIENTED_EDGE ( 'NONE', *, *, #25117, .T. ) ;
#41268=VERTEX_POINT ( 'NONE', #43464 ) ;
#41270=LINE ( 'NONE', #10030, #20169 ) ;
#41277=AXIS2_PLACEMENT_3D ( 'NONE', #33748, #27381, #24401 ) ;
#41326=VERTEX_POINT ( 'NONE', #33170 ) ;
#41341=VERTEX_POINT ( 'NONE', #9029 ) ;
#41354=CARTESIAN_POINT ( 'NONE',  ( 59.92024162955036104, -14.76985142791844829, -18.18981465713234158 ) ) ;
#41359=CARTESIAN_POINT ( 'NONE',  ( 59.06582835810969812, -15.05120494781123597, -18.19321520033831519 ) ) ;
#41376=ORIENTED_EDGE ( 'NONE', *, *, #34063, .F. ) ;
#41396=CARTESIAN_POINT ( 'NONE',  ( -2.519837040009542228, -7.040662428133670048, -19.27661969603944669 ) ) ;
#41421=ORIENTED_EDGE ( 'NONE', *, *, #7045, .F. ) ;
#41433=CARTESIAN_POINT ( 'NONE',  ( 66.83296847043716582, 0.3323961765722378003, -8.951213684657119529 ) ) ;
#41453=B_SPLINE_CURVE_WITH_KNOTS ( 'NONE', 3,
 ( #4903, #18819, #14954, #32710, #39795, #8564, #5129, #19046, #28866, #21569, #32933, #1708, #35456, #32044, #11540, #40019 ),
 .UNSPECIFIED., .F., .F.,
 ( 4, 2, 2, 2, 2, 2, 2, 4 ),
 ( 6.992893892674702526E-18, 0.001905203037969943657, 0.002857804556954912124, 0.003810406075939880375, 0.004763007594924848626, 0.005715609113909817310, 0.006668210632894785127, 0.007620812151879753811 ),
 .UNSPECIFIED. ) ;
#41467=EDGE_CURVE ( 'NONE', #39048, #26194, #28159, .T. ) ;
#41494=EDGE_CURVE ( 'NONE', #166, #5970, #36101, .T. ) ;
#41505=ORIENTED_EDGE ( 'NONE', *, *, #15842, .T. ) ;
#41512=ORIENTED_EDGE ( 'NONE', *, *, #39891, .T. ) ;
#41529=ORIENTED_EDGE ( 'NONE', *, *, #32432, .F. ) ;
#41545=AXIS2_PLACEMENT_3D ( 'NONE', #32, #21004, #34879 ) ;
#41551=FACE_OUTER_BOUND ( 'NONE', #23878, .T. ) ;
#41558=ORIENTED_EDGE ( 'NONE', *, *, #20384, .T. ) ;
#41578=VECTOR ( 'NONE', #36552, 1000.000000000000000 ) ;
#41588=ORIENTED_EDGE ( 'NONE', *, *, #15156, .F. ) ;
#41602=CARTESIAN_POINT ( 'NONE',  ( 59.77099224207091055, -14.81899841792058226, -8.593215200338313764 ) ) ;
#41629=DIRECTION ( 'NONE',  ( 0.9489384314806882381, 0.3124801273375108490, -0.04326688431241968585 ) ) ;
#41653=CARTESIAN_POINT ( 'NONE',  ( 62.78991778472225604, -1.552662796812879664, -7.442402790401765778 ) ) ;
#41700=CARTESIAN_POINT ( 'NONE',  ( 61.05647571779960003, -46.63990697477660063, -14.39321520033831625 ) ) ;
#41707=( BOUNDED_CURVE ( )  B_SPLINE_CURVE ( 3, ( #16928, #19487, #41105, #7096 ),
 .UNSPECIFIED., .F., .F. ) 
 B_SPLINE_CURVE_WITH_KNOTS ( ( 4, 4 ),
 ( 0.000000000000000000, 1.570796326794895004 ),
 .UNSPECIFIED. ) 
 CURVE ( )  GEOMETRIC_REPRESENTATION_ITEM ( )  RATIONAL_B_SPLINE_CURVE ( ( 1.000000000000000000, 0.8047378541243659367, 0.8047378541243659367, 1.000000000000000000 ) ) 
 REPRESENTATION_ITEM ( '' )  );
#41710=DIRECTION ( 'NONE',  ( 0.000000000000000000, 0.000000000000000000, -1.000000000000000000 ) ) ;
#41711=VECTOR ( 'NONE', #2239, 1000.000000000000000 ) ;
#41717=B_SPLINE_CURVE_WITH_KNOTS ( 'NONE', 3,
 ( #1527, #22289, #43268, #25266, #4505, #12034, #18427, #25936, #22508, #42372, #19088, #11133, #7699, #38928, #11582, #32319, #1084, #14998, #24269, #3279, #26385, #24046, #16756, #37939, #1978, #15674, #29803, #31094, #17202, #5402, #30652, #13336, #27240 ),
 .UNSPECIFIED., .F., .F.,
 ( 4, 2, 2, 2, 1, 1, 1, 1, 2, 2, 2, 2, 1, 1, 1, 1, 1, 2, 2, 2, 4 ),
 ( 0.000000000000000000, 0.2500000000003253509, 0.3750000000004861112, 0.4375000000005684342, 0.4687500000006095124, 0.4843750000006301071, 0.4921875000006404322, 0.4960937500006456502, 0.4980468750006464274, 0.5000000000006471490, 0.6250000000005297984, 0.6875000000004711787, 0.7187500000004417577, 0.7343750000004271028, 0.7421875000004197753, 0.7460937500004142242, 0.7480468750004114487, 0.7490234375004118927, 0.7500000000004123368, 0.8750000000002061684, 1.000000000000000000 ),
 .UNSPECIFIED. ) ;
#41731=CARTESIAN_POINT ( 'NONE',  ( 59.36680634945872725, -12.84644995903807896, -17.39321520033831447 ) ) ;
#41746=EDGE_CURVE ( 'NONE', #38238, #24192, #11951, .T. ) ;
#41768=DIRECTION ( 'NONE',  ( 0.9908103287288504424, -0.1352586133457950590, 0.000000000000000000 ) ) ;
#41830=ORIENTED_EDGE ( 'NONE', *, *, #16682, .T. ) ;
#41833=DIRECTION ( 'NONE',  ( 0.9063289528979890930, 0.4225728684367167087, 0.000000000000000000 ) ) ;
#41850=LINE ( 'NONE', #10610, #11639 ) ;
#41876=CARTESIAN_POINT ( 'NONE',  ( 64.08833547316721990, -12.91438983140282559, -15.87665273277405831 ) ) ;
#41877=CARTESIAN_POINT ( 'NONE',  ( 67.19031194842951038, -1.707697914625855296, -14.39321520033831625 ) ) ;
#41890=( BOUNDED_SURFACE ( )  B_SPLINE_SURFACE ( 3, 2, ( 
 ( #20143, #44988, #23792 ),
 ( #41354, #26752, #40659 ),
 ( #10110, #13747, #23567 ),
 ( #44316, #24014, #37902 ) ),
 .UNSPECIFIED., .F., .F., .T. ) 
 B_SPLINE_SURFACE_WITH_KNOTS ( ( 4, 4 ),
 ( 3, 3 ),
 ( 1.522649623061655300, 1.570796326794896558 ),
 ( 0.000000000000000000, 1.000000000000000000 ),
 .UNSPECIFIED. ) 
 GEOMETRIC_REPRESENTATION_ITEM ( )  RATIONAL_B_SPLINE_SURFACE ( (
 ( 1.000000000000000000, 0.7145271066604789167, 1.000000000000000000),
 ( 1.000000000000000000, 0.7120684114869153536, 1.000000000000000000),
 ( 1.000000000000000000, 0.7095941637304922223, 1.000000000000000000),
 ( 1.000000000000000000, 0.7071067811865475727, 1.000000000000000000) ) ) 
 REPRESENTATION_ITEM ( '' )  SURFACE ( )  );
#41905=ORIENTED_EDGE ( 'NONE', *, *, #32827, .F. ) ;
#41910=EDGE_CURVE ( 'NONE', #42200, #26749, #36366, .T. ) ;
#41919=DIRECTION ( 'NONE',  ( 0.000000000000000000, 0.000000000000000000, -1.000000000000000000 ) ) ;
#41943=DIRECTION ( 'NONE',  ( 0.9986099732815399976, 0.05270788615228315377, 0.000000000000000000 ) ) ;
#41952=CARTESIAN_POINT ( 'NONE',  ( 60.51499503671957569, -14.57400245158741114, -18.15781989776658989 ) ) ;
#41963=LINE ( 'NONE', #13706, #32957 ) ;
#41972=ORIENTED_EDGE ( 'NONE', *, *, #12819, .F. ) ;
#41978=ORIENTED_EDGE ( 'NONE', *, *, #9793, .T. ) ;
#41983=DIRECTION ( 'NONE',  ( -0.9908103287288503314, 0.1352586133457956419, 0.000000000000000000 ) ) ;
#42009=CARTESIAN_POINT ( 'NONE',  ( 62.83933201006748703, -13.37155033267121595, -18.76174004378365012 ) ) ;
#42012=ORIENTED_EDGE ( 'NONE', *, *, #16982, .F. ) ;
#42026=DIRECTION ( 'NONE',  ( -0.7962509850245453880, -0.6049664196031389052, 0.000000000000000000 ) ) ;
#42046=EDGE_CURVE ( 'NONE', #39949, #166, #26075, .T. ) ;
#42050=ADVANCED_FACE ( 'NONE', ( #31068 ), #34475, .T. ) ;
#42052=ORIENTED_EDGE ( 'NONE', *, *, #17527, .T. ) ;
#42064=VECTOR ( 'NONE', #16996, 1000.000000000000000 ) ;
#42066=CARTESIAN_POINT ( 'NONE',  ( 63.92618626571611173, -15.01321783771253138, -16.50148821192263426 ) ) ;
#42096=CARTESIAN_POINT ( 'NONE',  ( 71.99789814782840836, -24.87091310681484657, -7.393215200338315363 ) ) ;
#42099=CARTESIAN_POINT ( 'NONE',  ( -12.36826994950264336, -4.374949827406453551, -7.393215200338315363 ) ) ;
#42110=EDGE_LOOP ( 'NONE', ( #20101, #8235, #40865, #29629, #9653, #41421, #1195, #43454 ) ) ;
#42123=DIRECTION ( 'NONE',  ( -0.9908103287288505534, 0.1352586133457944206, 0.000000000000000000 ) ) ;
#42145=DIRECTION ( 'NONE',  ( 0.9908103287288505534, -0.1352586133457944206, 0.000000000000000000 ) ) ;
#42150=CARTESIAN_POINT ( 'NONE',  ( 60.53937939559665438, -4.256997083809236138, -7.393215200338315363 ) ) ;
#42166=LINE ( 'NONE', #35752, #31373 ) ;
#42168=AXIS2_PLACEMENT_3D ( 'NONE', #1293, #5155, #15205 ) ;
#42175=CARTESIAN_POINT ( 'NONE',  ( 64.85962650386538542, -13.90972770790538071, -17.69353582949934278 ) ) ;
#42178=DIRECTION ( 'NONE',  ( 0.000000000000000000, 0.000000000000000000, -1.000000000000000000 ) ) ;
#42179=ORIENTED_EDGE ( 'NONE', *, *, #401, .F. ) ;
#42185=CARTESIAN_POINT ( 'NONE',  ( 0.000000000000000000, 0.000000000000000000, 0.000000000000000000 ) ) ;
#42188=DIRECTION ( 'NONE',  ( 0.000000000000000000, 0.000000000000000000, -1.000000000000000000 ) ) ;
#42200=VERTEX_POINT ( 'NONE', #9654 ) ;
#42202=VECTOR ( 'NONE', #31045, 1000.000000000000000 ) ;
#42206=CARTESIAN_POINT ( 'NONE',  ( 59.44377208703740223, -12.82110557137145967, -9.393546723914594665 ) ) ;
#42218=CARTESIAN_POINT ( 'NONE',  ( 69.69189222815028018, -41.76310523276638520, -10.89321520033831447 ) ) ;
#42225=VERTEX_POINT ( 'NONE', #3254 ) ;
#42255=ORIENTED_EDGE ( 'NONE', *, *, #14170, .T. ) ;
#42277=CIRCLE ( 'NONE', #25516, 4.999999999999998224 ) ;
#42287=EDGE_LOOP ( 'NONE', ( #43425, #41075, #9504, #23680 ) ) ;
#42291=CARTESIAN_POINT ( 'NONE',  ( 64.48003408175695483, -13.07484350022234132, -11.22706228626448421 ) ) ;
#42313=CARTESIAN_POINT ( 'NONE',  ( 64.21381391893872603, -15.17632890891775510, -10.58270692696840598 ) ) ;
#42323=FACE_OUTER_BOUND ( 'NONE', #15158, .T. ) ;
#42354=ORIENTED_EDGE ( 'NONE', *, *, #10663, .T. ) ;
#42363=AXIS2_PLACEMENT_3D ( 'NONE', #22378, #18740, #35821 ) ;
#42366=ORIENTED_EDGE ( 'NONE', *, *, #18903, .T. ) ;
#42372=CARTESIAN_POINT ( 'NONE',  ( 64.81879891447307784, -2.621774883878052353, -8.236146696172697901 ) ) ;
#42398=CARTESIAN_POINT ( 'NONE',  ( 62.93948576833484054, -14.63887389195935107, -17.26917803626528780 ) ) ;
#42406=CARTESIAN_POINT ( 'NONE',  ( 67.19031194842951038, -1.707697914625855296, -12.39321520033831447 ) ) ;
#42420=EDGE_CURVE ( 'NONE', #41268, #33252, #430, .T. ) ;
#42421=( BOUNDED_CURVE ( )  B_SPLINE_CURVE ( 3, ( #42206, #21225, #38532, #10308 ),
 .UNSPECIFIED., .F., .T. ) 
 B_SPLINE_CURVE_WITH_KNOTS ( ( 4, 4 ),
 ( 4.703285054500009998, 4.712388980384689674 ),
 .UNSPECIFIED. ) 
 CURVE ( )  GEOMETRIC_REPRESENTATION_ITEM ( )  RATIONAL_B_SPLINE_CURVE ( ( 1.000000000000000000, 0.9999930932230500780, 0.9999930932230500780, 1.000000000000000000 ) ) 
 REPRESENTATION_ITEM ( '' )  );
#42439=CARTESIAN_POINT ( 'NONE',  ( 75.95778847736514194, -3.256761025687008537, -14.39321520033831625 ) ) ;
#42455=CARTESIAN_POINT ( 'NONE',  ( 64.76452260854004805, -13.87123648633731854, -17.75937495128697918 ) ) ;
#42460=VERTEX_POINT ( 'NONE', #22153 ) ;
#42463=AXIS2_PLACEMENT_3D ( 'NONE', #31116, #13130, #37505 ) ;
#42487=ORIENTED_EDGE ( 'NONE', *, *, #40126, .T. ) ;
#42492=CIRCLE ( 'NONE', #5340, 6.999999999999999112 ) ;
#42549=CARTESIAN_POINT ( 'NONE',  ( 63.69959400472163935, -14.91280095328349020, -10.08899308684463847 ) ) ;
#42594=CARTESIAN_POINT ( 'NONE',  ( -13.78096647419814680, -4.499153416623470569, -8.147705117616510506 ) ) ;
#42613=ORIENTED_EDGE ( 'NONE', *, *, #43534, .T. ) ;
#42617=CARTESIAN_POINT ( 'NONE',  ( 63.43088374006683239, -46.96404483173760269, -16.39321520033831447 ) ) ;
#42623=CARTESIAN_POINT ( 'NONE',  ( -13.52853001603108574, -4.831407855809472629, -18.06453541021588194 ) ) ;
#42624=FACE_OUTER_BOUND ( 'NONE', #26033, .T. ) ;
#42635=DIRECTION ( 'NONE',  ( 0.9908103287288655414, -0.1352586133456837314, 0.000000000000000000 ) ) ;
#42637=ORIENTED_EDGE ( 'NONE', *, *, #44678, .F. ) ;
#42640=CARTESIAN_POINT ( 'NONE',  ( 63.42519601278144847, -3.154277804759124226, -19.11392337093018767 ) ) ;
#42641=ORIENTED_EDGE ( 'NONE', *, *, #4454, .T. ) ;
#42644=CIRCLE ( 'NONE', #6224, 1.500000000000000000 ) ;
#42650=CARTESIAN_POINT ( 'NONE',  ( 60.34146317132753978, -13.36775875599912844, -18.19321520033831519 ) ) ;
#42655=CARTESIAN_POINT ( 'NONE',  ( 31.16203868753470019, 11.28474725185576055, -17.89321520033831447 ) ) ;
#42695=VECTOR ( 'NONE', #8301, 1000.000000000000000 ) ;
#42709=EDGE_CURVE ( 'NONE', #30504, #19352, #12132, .T. ) ;
#42713=DIRECTION ( 'NONE',  ( 0.000000000000000000, 0.000000000000000000, -1.000000000000000000 ) ) ;
#42720=DIRECTION ( 'NONE',  ( -0.000000000000000000, 0.000000000000000000, 1.000000000000000000 ) ) ;
#42724=CARTESIAN_POINT ( 'NONE',  ( 75.95778847736514194, -3.256761025687008537, -14.39321520033831625 ) ) ;
#42726=EDGE_CURVE ( 'NONE', #511, #43799, #19182, .T. ) ;
#42727=CIRCLE ( 'NONE', #41277, 5.500000000000001776 ) ;
#42748=DIRECTION ( 'NONE',  ( 0.1352586133457954198, 0.9908103287288503314, 0.000000000000000000 ) ) ;
#42765=DIRECTION ( 'NONE',  ( 0.000000000000000000, 0.000000000000000000, 1.000000000000000000 ) ) ;
#42778=CARTESIAN_POINT ( 'NONE',  ( 61.65126288137282273, -14.46472726967718181, -8.900850585800878179 ) ) ;
#42783=VERTEX_POINT ( 'NONE', #29438 ) ;
#42820=DIRECTION ( 'NONE',  ( -0.3127730236694426513, 0.9498278979187093629, 0.000000000000000000 ) ) ;
#42824=CARTESIAN_POINT ( 'NONE',  ( 66.03584176102988579, -0.1449045395527848445, -16.39321520033830737 ) ) ;
#42848=CARTESIAN_POINT ( 'NONE',  ( 63.48709602856936129, -14.78504216833964335, -18.40560711939649252 ) ) ;
#42860=( NAMED_UNIT ( * ) PLANE_ANGLE_UNIT ( ) SI_UNIT ( $, .RADIAN. ) );
#42864=CARTESIAN_POINT ( 'NONE',  ( 66.07631794059973629, -2.141239331173074856, -18.04181533358571343 ) ) ;
#42866=EDGE_CURVE ( 'NONE', #18085, #24134, #13025, .T. ) ;
#42868=EDGE_CURVE ( 'NONE', #6119, #31347, #42727, .T. ) ;
#42879=DIRECTION ( 'NONE',  ( -0.9063289528979890930, -0.4225728684367167087, 0.000000000000000000 ) ) ;
#42880=VECTOR ( 'NONE', #30511, 1000.000000000000000 ) ;
#42881=CARTESIAN_POINT ( 'NONE',  ( 80.91184012100937650, -3.933054092416038650, -19.39321520033831447 ) ) ;
#42899=CARTESIAN_POINT ( 'NONE',  ( 80.91184012100937650, -3.933054092416038650, -10.89321520033831447 ) ) ;
#42918=CARTESIAN_POINT ( 'NONE',  ( 65.41257106814472877, -15.47412461924279725, -10.39321520033831625 ) ) ;
#42927=EDGE_LOOP ( 'NONE', ( #28521, #8005, #39724, #1292 ) ) ;
#42933=LINE ( 'NONE', #24478, #25705 ) ;
#42941=CARTESIAN_POINT ( 'NONE',  ( 60.45894907855898026, -4.846173528048905332, -19.39321520033831447 ) ) ;
#42993=CARTESIAN_POINT ( 'NONE',  ( 63.13932362937020315, -14.69787538488875533, -9.650383735752717129 ) ) ;
#43038=CARTESIAN_POINT ( 'NONE',  ( -13.67905184926989826, -4.633292466094534490, -7.903589911137905766 ) ) ;
#43042=CARTESIAN_POINT ( 'NONE',  ( 67.90996757083897251, -0.5187677644655397380, -16.39321520033831447 ) ) ;
#43085=CARTESIAN_POINT ( 'NONE',  ( 60.53937939559665438, -4.256997083809236138, -19.39321520033831447 ) ) ;
#43127=DIRECTION ( 'NONE',  ( -0.9063289528979876497, -0.4225728684367200394, 0.000000000000000000 ) ) ;
#43135=CIRCLE ( 'NONE', #25656, 1.199999999999999512 ) ;
#43137=VECTOR ( 'NONE', #3898, 1000.000000000000000 ) ;
#43140=VERTEX_POINT ( 'NONE', #10133 ) ;
#43146=ORIENTED_EDGE ( 'NONE', *, *, #42866, .F. ) ;
#43155=FACE_OUTER_BOUND ( 'NONE', #30280, .T. ) ;
#43183=CARTESIAN_POINT ( 'NONE',  ( 62.47183387988239645, -3.518612362980701125, -19.22720551556120228 ) ) ;
#43212=CARTESIAN_POINT ( 'NONE',  ( 75.95778847736514194, -3.256761025687008537, -7.147228641687434880 ) ) ;
#43215=CARTESIAN_POINT ( 'NONE',  ( 64.37417719139408234, -13.02885965268791324, -15.64938273518901291 ) ) ;
#43216=DIRECTION ( 'NONE',  ( 0.1352586133457950590, 0.9908103287288504424, 1.214306433183764177E-14 ) ) ;
#43222=CARTESIAN_POINT ( 'NONE',  ( 65.34866896724287244, -14.13234089959629536, -9.463491280356649327 ) ) ;
#43225=ORIENTED_EDGE ( 'NONE', *, *, #40636, .T. ) ;
#43231=AXIS2_PLACEMENT_3D ( 'NONE', #34096, #9950, #9040 ) ;
#43268=CARTESIAN_POINT ( 'NONE',  ( 67.18677111376662481, -1.717760636639239280, -9.553179424549121279 ) ) ;
#43269=LINE ( 'NONE', #18863, #22357 ) ;
#43294=CARTESIAN_POINT ( 'NONE',  ( -13.56828337869051460, -4.779084862086333096, -17.94035226225507884 ) ) ;
#43296=PLANE ( 'NONE',  #34812 ) ;
#43297=TOROIDAL_SURFACE ( 'NONE', #17106, 4.500000000000000000, 0.5000000000000000000 ) ;
#43299=ORIENTED_EDGE ( 'NONE', *, *, #43431, .T. ) ;
#43323=ADVANCED_BREP_SHAPE_REPRESENTATION ( '', ( #21433, #12375 ), #19397 ) ;
#43325=VECTOR ( 'NONE', #18814, 1000.000000000000000 ) ;
#43371=EDGE_LOOP ( 'NONE', ( #7292, #20946, #24633, #5319 ) ) ;
#43376=CARTESIAN_POINT ( 'NONE',  ( 65.52066458535989568, -15.46830930983349184, -16.39321520033831092 ) ) ;
#43377=ADVANCED_FACE ( 'NONE', ( #13770 ), #10572, .T. ) ;
#43379=DIRECTION ( 'NONE',  ( -0.000000000000000000, -0.000000000000000000, 1.000000000000000000 ) ) ;
#43387=CARTESIAN_POINT ( 'NONE',  ( 75.95778847736514194, -3.256761025687008537, -19.39321520033831447 ) ) ;
#43418=ORIENTED_EDGE ( 'NONE', *, *, #13240, .T. ) ;
#43425=ORIENTED_EDGE ( 'NONE', *, *, #7215, .T. ) ;
#43431=EDGE_CURVE ( 'NONE', #39048, #41341, #31096, .T. ) ;
#43442=CARTESIAN_POINT ( 'NONE',  ( 64.38259412312832808, -13.03244878199202361, -15.64233727451349054 ) ) ;
#43448=TOROIDAL_SURFACE ( 'NONE', #512, 6.500000000000000000, 1.500000000000000000 ) ;
#43449=CARTESIAN_POINT ( 'NONE',  ( 65.49030871267177645, -0.3060001693188343919, -10.39321520033831447 ) ) ;
#43450=CARTESIAN_POINT ( 'NONE',  ( -2.329871626679969054, -6.983709645767248730, -19.17689330043476659 ) ) ;
#43451=CARTESIAN_POINT ( 'NONE',  ( 60.62026699881264591, -14.54430726831175669, -7.482851213058667739 ) ) ;
#43454=ORIENTED_EDGE ( 'NONE', *, *, #25101, .F. ) ;
#43456=CARTESIAN_POINT ( 'NONE',  ( 65.83110444452054821, -15.38354445881851440, -10.39321520033831625 ) ) ;
#43464=CARTESIAN_POINT ( 'NONE',  ( -6.962123463324038752, -11.49046785505262669, -7.393215200338315363 ) ) ;
#43466=CARTESIAN_POINT ( 'NONE',  ( -13.56828337869050927, -4.779084862086334873, -8.893215200338314474 ) ) ;
#43468=CARTESIAN_POINT ( 'NONE',  ( -12.36826994950264336, -4.374949827406451774, -19.39321520033831803 ) ) ;
#43477=EDGE_CURVE ( 'NONE', #13151, #26347, #32192, .T. ) ;
#43520=ORIENTED_EDGE ( 'NONE', *, *, #2147, .F. ) ;
#43526=ORIENTED_EDGE ( 'NONE', *, *, #24911, .T. ) ;
#43531=CARTESIAN_POINT ( 'NONE',  ( 42.57150613532612482, -13.18613447638990088, -12.39321520033831447 ) ) ;
#43534=EDGE_CURVE ( 'NONE', #3183, #31639, #21111, .T. ) ;
#43598=ADVANCED_FACE ( 'NONE', ( #36059 ), #24566, .T. ) ;
#43650=CARTESIAN_POINT ( 'NONE',  ( 67.08264006073221708, -20.21382323020432992, -15.89321520033831447 ) ) ;
#43655=AXIS2_PLACEMENT_3D ( 'NONE', #39866, #15470, #15698 ) ;
#43660=VERTEX_POINT ( 'NONE', #35608 ) ;
#43664=CARTESIAN_POINT ( 'NONE',  ( 71.31713442278437753, 2.423123680056944007, -10.89321520033831447 ) ) ;
#43672=FACE_OUTER_BOUND ( 'NONE', #27247, .T. ) ;
#43684=CARTESIAN_POINT ( 'NONE',  ( -13.78505786849313886, -3.796669023460156556, -17.89321520033824697 ) ) ;
#43715=LINE ( 'NONE', #16814, #8749 ) ;
#43717=LINE ( 'NONE', #15221, #44222 ) ;
#43720=CARTESIAN_POINT ( 'NONE',  ( 67.59280524186679884, -0.2640895998874671635, -16.39321520033831447 ) ) ;
#43721=DIRECTION ( 'NONE',  ( -0.9908103287288504424, 0.1352586133457951423, 0.000000000000000000 ) ) ;
#43799=VERTEX_POINT ( 'NONE', #30701 ) ;
#43824=ORIENTED_EDGE ( 'NONE', *, *, #5061, .T. ) ;
#43834=CARTESIAN_POINT ( 'NONE',  ( 66.50565249108366572, -35.53029877516337365, -14.39321520033831625 ) ) ;
#43858=CARTESIAN_POINT ( 'NONE',  ( 67.18674234710391602, -1.717770130243481574, -17.23327264932555281 ) ) ;
#43861=CARTESIAN_POINT ( 'NONE',  ( -3.049798262687883010, -7.199197394943047890, -7.393215200338317139 ) ) ;
#43879=ORIENTED_EDGE ( 'NONE', *, *, #23426, .T. ) ;
#43886=FACE_OUTER_BOUND ( 'NONE', #938, .T. ) ;
#43891=CARTESIAN_POINT ( 'NONE',  ( 81.31761596104672662, -0.9606231062294252609, -12.39321520033831447 ) ) ;
#43900=CARTESIAN_POINT ( 'NONE',  ( 67.40573139832108041, -0.1776877719995537119, -10.39321520033831625 ) ) ;
#43901=CARTESIAN_POINT ( 'NONE',  ( -2.802086886829308732, -7.125079315770471489, -19.36905904446185289 ) ) ;
#43917=CARTESIAN_POINT ( 'NONE',  ( -12.68878346039663363, -4.256507409708595091, -19.36568748919502880 ) ) ;
#43952=CIRCLE ( 'NONE', #3900, 11.00000000000000000 ) ;
#43961=DIRECTION ( 'NONE',  ( -0.9908103287288504424, 0.1352586133457950868, 0.000000000000000000 ) ) ;
#43977=ORIENTED_EDGE ( 'NONE', *, *, #36192, .T. ) ;
#43987=EDGE_CURVE ( 'NONE', #18085, #1795, #6304, .T. ) ;
#43998=DIRECTION ( 'NONE',  ( 0.05270788615228318846, -0.9986099732815399976, 2.696077241641140828E-16 ) ) ;
#44000=VERTEX_POINT ( 'NONE', #21098 ) ;
#44042=DIRECTION ( 'NONE',  ( -0.9498278979187094739, -0.3127730236694427068, -0.000000000000000000 ) ) ;
#44054=AXIS2_PLACEMENT_3D ( 'NONE', #22012, #11535, #38878 ) ;
#44061=CARTESIAN_POINT ( 'NONE',  ( 66.16802772684418699, -15.11730172789017423, -16.39321520033831447 ) ) ;
#44089=CARTESIAN_POINT ( 'NONE',  ( 62.57128181610967488, -3.480577623552236766, -19.20948089883370713 ) ) ;
#44093=CARTESIAN_POINT ( 'NONE',  ( 31.33087284928346605, -19.31933043625826230, -8.593215200338315540 ) ) ;
#44095=CARTESIAN_POINT ( 'NONE',  ( -1.667125314829374982, -6.784308280680000358, -8.532095462264171815 ) ) ;
#44123=B_SPLINE_CURVE_WITH_KNOTS ( 'NONE', 3,
 ( #257, #21011, #25780, #36476, #4343, #39687 ),
 .UNSPECIFIED., .F., .F.,
 ( 4, 2, 4 ),
 ( -8.394000326495523731E-06, 0.0005522989975109767087, 0.001112991995348449085 ),
 .UNSPECIFIED. ) ;
#44124=DIRECTION ( 'NONE',  ( -0.9908103287288505534, 0.1352586133457944206, 0.000000000000000000 ) ) ;
#44132=LINE ( 'NONE', #15629, #29361 ) ;
#44136=AXIS2_PLACEMENT_3D ( 'NONE', #26808, #9708, #2622 ) ;
#44146=AXIS2_PLACEMENT_3D ( 'NONE', #15281, #4788, #1144 ) ;
#44212=LINE ( 'NONE', #16848, #42880 ) ;
#44222=VECTOR ( 'NONE', #39622, 1000.000000000000000 ) ;
#44240=ADVANCED_FACE ( 'NONE', ( #38702 ), #29172, .T. ) ;
#44249=CIRCLE ( 'NONE', #10748, 0.5000000000000004441 ) ;
#44257=CARTESIAN_POINT ( 'NONE',  ( 27.57768543387103222, -14.97172645945875935, -7.393215200338315363 ) ) ;
#44275=DIRECTION ( 'NONE',  ( 0.3127730236694426513, -0.9498278979187093629, 0.000000000000000000 ) ) ;
#44280=EDGE_CURVE ( 'NONE', #31011, #43660, #18738, .T. ) ;
#44284=ORIENTED_EDGE ( 'NONE', *, *, #44897, .F. ) ;
#44316=CARTESIAN_POINT ( 'NONE',  ( 59.62174278132244609, -14.86814543204979522, -18.19321520033831874 ) ) ;
#44319=CARTESIAN_POINT ( 'NONE',  ( 62.51884409362852324, -3.500628399893147336, -19.21898247060032006 ) ) ;
#44322=DIRECTION ( 'NONE',  ( 0.9498278979187092519, 0.3127730236694430399, -0.000000000000000000 ) ) ;
#44324=CARTESIAN_POINT ( 'NONE',  ( -1.637506834317629112, -6.775152287193631828, -8.718355983560822864 ) ) ;
#44332=ORIENTED_EDGE ( 'NONE', *, *, #7095, .F. ) ;
#44337=EDGE_LOOP ( 'NONE', ( #3269, #15132, #15589, #8903 ) ) ;
#44338=EDGE_CURVE ( 'NONE', #3386, #5770, #41717, .T. ) ;
#44368=CARTESIAN_POINT ( 'NONE',  ( 59.69399050597295542, -13.58096788970640567, -18.18301750815651374 ) ) ;
#44426=CARTESIAN_POINT ( 'NONE',  ( 41.72636039845269096, -11.37347657059392070, -8.893215200338314474 ) ) ;
#44447=ORIENTED_EDGE ( 'NONE', *, *, #20334, .F. ) ;
#44454=LINE ( 'NONE', #26666, #29619 ) ;
#44491=CARTESIAN_POINT ( 'NONE',  ( 80.41643495664496299, -3.865424785743139857, -15.89321520033831447 ) ) ;
#44502=CARTESIAN_POINT ( 'NONE',  ( 61.93073106961468000, -12.47488654111867312, -9.789137930298094759 ) ) ;
#44510=DIRECTION ( 'NONE',  ( -0.1352586133457950590, -0.9908103287288504424, 0.000000000000000000 ) ) ;
#44526=AXIS2_PLACEMENT_3D ( 'NONE', #8086, #14927, #8982 ) ;
#44561=ADVANCED_FACE ( 'NONE', ( #35622 ), #14218, .T. ) ;
#44568=ORIENTED_EDGE ( 'NONE', *, *, #33629, .F. ) ;
#44586=DIRECTION ( 'NONE',  ( -0.9063289528979890930, -0.4225728684367167087, 0.000000000000000000 ) ) ;
#44599=DIRECTION ( 'NONE',  ( 0.000000000000000000, 0.000000000000000000, -1.000000000000000000 ) ) ;
#44627=ADVANCED_FACE ( 'NONE', ( #43155 ), #16488, .T. ) ;
#44642=DIRECTION ( 'NONE',  ( 0.000000000000000000, 0.000000000000000000, 1.000000000000000000 ) ) ;
#44666=AXIS2_PLACEMENT_3D ( 'NONE', #5786, #12199, #40692 ) ;
#44678=EDGE_CURVE ( 'NONE', #18111, #33252, #21551, .T. ) ;
#44683=CIRCLE ( 'NONE', #22075, 8.800000000000000711 ) ;
#44692=EDGE_CURVE ( 'NONE', #2818, #44000, #37567, .T. ) ;
#44724=CYLINDRICAL_SURFACE ( 'NONE', #30765, 0.5000000000000038858 ) ;
#44727=ORIENTED_EDGE ( 'NONE', *, *, #4240, .F. ) ;
#44747=DIRECTION ( 'NONE',  ( 0.4225728684367167087, -0.9063289528979890930, -0.000000000000000000 ) ) ;
#44772=AXIS2_PLACEMENT_3D ( 'NONE', #4613, #1199, #15334 ) ;
#44795=CARTESIAN_POINT ( 'NONE',  ( 59.62174278132244609, -14.86814543204979522, -8.593215200338313764 ) ) ;
#44809=DIRECTION ( 'NONE',  ( 0.000000000000000000, 0.000000000000000000, -1.000000000000000000 ) ) ;
#44815=DIRECTION ( 'NONE',  ( 0.000000000000000000, 0.000000000000000000, 1.000000000000000000 ) ) ;
#44828=CARTESIAN_POINT ( 'NONE',  ( 74.47157298427187300, -3.053873105668316601, -7.147228641687434880 ) ) ;
#44850=DIRECTION ( 'NONE',  ( -0.9063289528979890930, -0.4225728684367167087, 0.000000000000000000 ) ) ;
#44874=CARTESIAN_POINT ( 'NONE',  ( 69.69189222815028018, -41.76310523276638520, -7.393215200338315363 ) ) ;
#44878=AXIS2_PLACEMENT_3D ( 'NONE', #10949, #28280, #35772 ) ;
#44879=CARTESIAN_POINT ( 'NONE',  ( 69.69189222815028018, -41.76310523276638520, -16.39321520033831447 ) ) ;
#44882=LINE ( 'NONE', #44426, #30588 ) ;
#44887=ORIENTED_EDGE ( 'NONE', *, *, #21494, .T. ) ;
#44897=EDGE_CURVE ( 'NONE', #22762, #42783, #27730, .T. ) ;
#44905=DIRECTION ( 'NONE',  ( -0.9908103287288505534, 0.1352586133457950035, 0.000000000000000000 ) ) ;
#44912=( BOUNDED_CURVE ( )  B_SPLINE_CURVE ( 3, ( #4447, #28184, #16298, #33365 ),
 .UNSPECIFIED., .F., .T. ) 
 B_SPLINE_CURVE_WITH_KNOTS ( ( 4, 4 ),
 ( 1.570796326794895004, 2.466461120652760020 ),
 .UNSPECIFIED. ) 
 CURVE ( )  GEOMETRIC_REPRESENTATION_ITEM ( )  RATIONAL_B_SPLINE_CURVE ( ( 1.000000000000000000, 0.9342585459106650392, 0.9342585459106650392, 1.000000000000000000 ) ) 
 REPRESENTATION_ITEM ( '' )  );
#44913=FACE_OUTER_BOUND ( 'NONE', #34427, .T. ) ;
#44953=VECTOR ( 'NONE', #44850, 1000.000000000000000 ) ;
#44958=CARTESIAN_POINT ( 'NONE',  ( 62.98033575700867459, -12.60074217725106394, -10.22254757083790722 ) ) ;
#44962=AXIS2_PLACEMENT_3D ( 'NONE', #19771, #29807, #43721 ) ;
#44970=LINE ( 'NONE', #1143, #3663 ) ;
#44988=CARTESIAN_POINT ( 'NONE',  ( 60.11760374155740294, -14.70486118635416695, -19.35686119223085555 ) ) ;
#45032=B_SPLINE_CURVE_WITH_KNOTS ( 'NONE', 3,
 ( #39344, #11082, #4672, #15170, #7881, #25665, #7648, #32485, #21789, #42099 ),
 .UNSPECIFIED., .F., .F.,
 ( 4, 2, 2, 2, 4 ),
 ( 0.000000000000000000, 0.0005979257515333403529, 0.001195851503066680706, 0.001793777254600021059, 0.002391703006133361412 ),
 .UNSPECIFIED. ) ;
#45071=CARTESIAN_POINT ( 'NONE',  ( 62.20960312368780620, -12.49232639468414163, -16.90032038405202997 ) ) ;
#45080=EDGE_LOOP ( 'NONE', ( #4795, #36590, #36902, #21460, #36898, #8991 ) ) ;
#45127=DIRECTION ( 'NONE',  ( 0.000000000000000000, 0.000000000000000000, 1.000000000000000000 ) ) ;
#45132=CIRCLE ( 'NONE', #16733, 4.500000000000000888 ) ;
#45156=COLOUR_RGB('Dark Blue',0.08,0.2,0.34);
#45157=FILL_AREA_STYLE_COLOUR('',#45156);
#45158=FILL_AREA_STYLE('',(#45157));
#45159=SURFACE_STYLE_FILL_AREA(#45158);
#45160=SURFACE_SIDE_STYLE('',(#45159));
#45161=SURFACE_STYLE_USAGE(.BOTH.,#45160);
#45162=PRESENTATION_STYLE_ASSIGNMENT((#45161));
ENDSEC;
END-ISO-10303-21;
